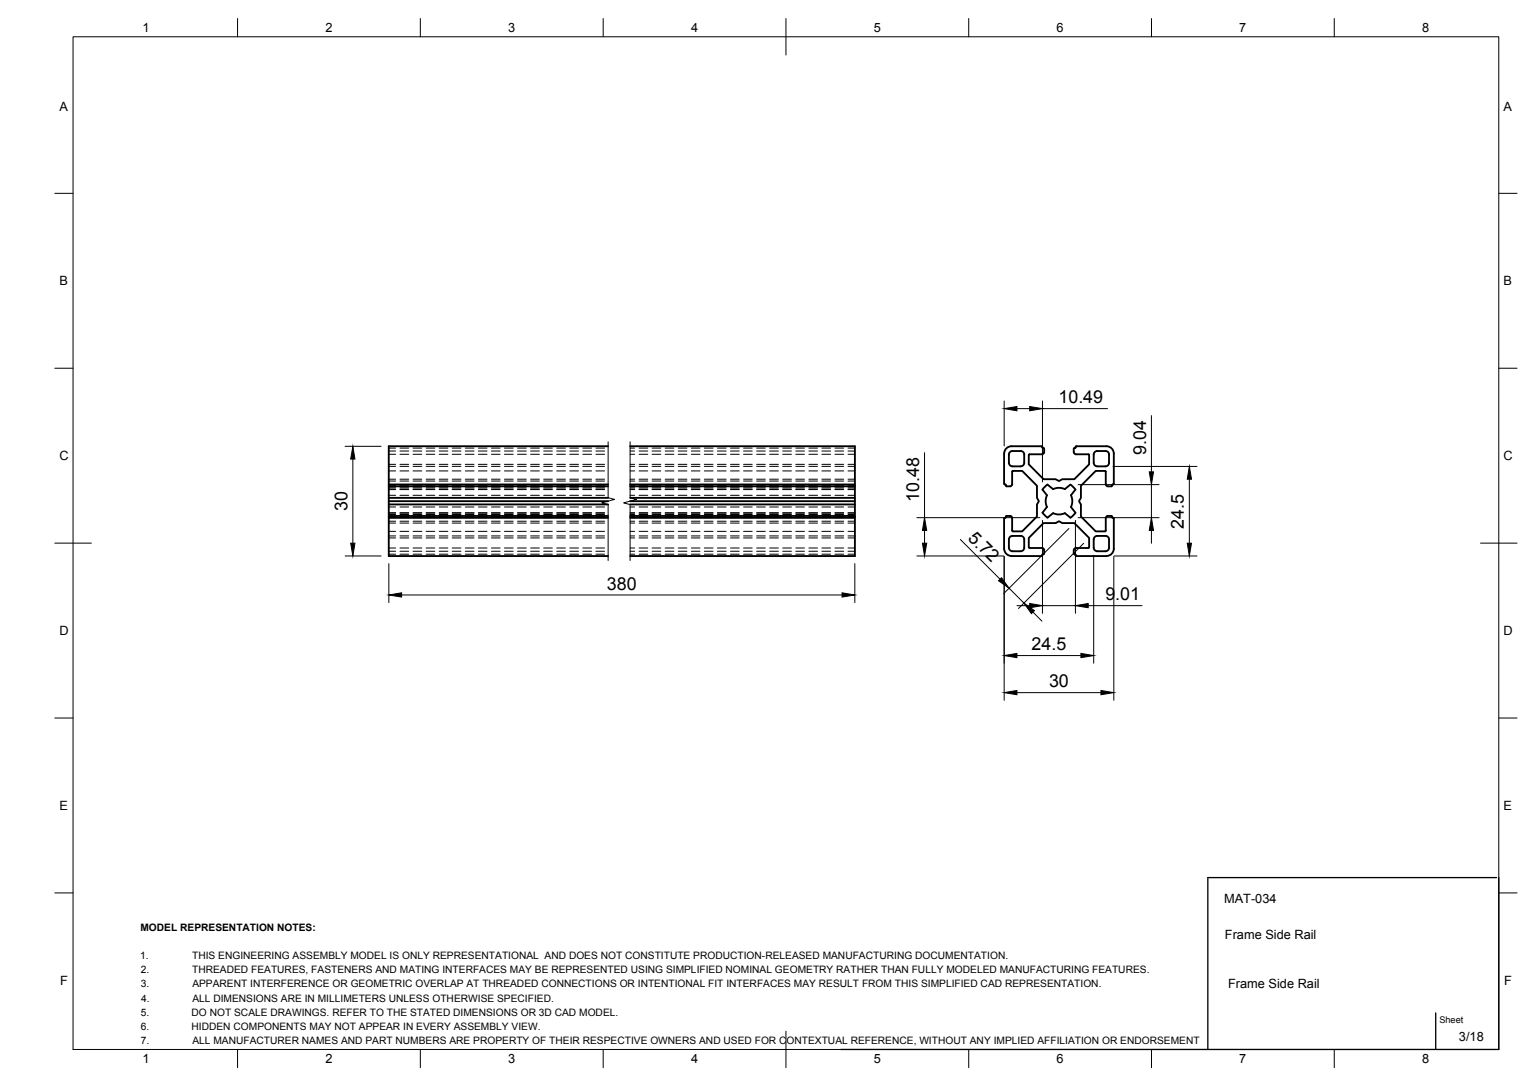
ISO-10303-21;
HEADER;
/* Generated by software containing ST-Developer
 * from STEP Tools, Inc. (www.steptools.com) 
 */

FILE_DESCRIPTION(
/* description */ ('STEP AP214'),
/* implementation_level */ '2;1');

FILE_NAME(
/* name */ 'Frame Side Rail.step',
/* time_stamp */ '2026-11-14T09:24:36-08:00',
/* author */ (''),
/* organization */ (''),
/* preprocessor_version */ 'ST-DEVELOPER v20.2',
/* originating_system */ 'Autodesk Translation Framework v15.17.0.0',
/* authorisation */ '');

FILE_SCHEMA (('AUTOMOTIVE_DESIGN { 1 0 10303 214 3 1 1 }'));
ENDSEC;

DATA;
#10=MECHANICAL_DESIGN_GEOMETRIC_PRESENTATION_REPRESENTATION('',(#213),#18867);
#181=SHAPE_REPRESENTATION_RELATIONSHIP('SRR','None',#18945,#197);
#197=ADVANCED_BREP_SHAPE_REPRESENTATION('',(#237),#18861);
#213=STYLED_ITEM('',(#19024),#237);
#237=MANIFOLD_SOLID_BREP('Body1',#10968);
#346=FACE_BOUND('',#1719,.T.);
#347=FACE_BOUND('',#1720,.T.);
#348=FACE_BOUND('',#1721,.T.);
#349=FACE_BOUND('',#1722,.T.);
#350=FACE_BOUND('',#1723,.T.);
#351=FACE_BOUND('',#1725,.T.);
#352=FACE_BOUND('',#1726,.T.);
#353=FACE_BOUND('',#1727,.T.);
#354=FACE_BOUND('',#1728,.T.);
#355=FACE_BOUND('',#1729,.T.);
#568=PLANE('',#11716);
#569=PLANE('',#11784);
#570=PLANE('',#11852);
#571=PLANE('',#11853);
#572=PLANE('',#11854);
#573=PLANE('',#11855);
#574=PLANE('',#11856);
#575=PLANE('',#11858);
#576=PLANE('',#11860);
#577=PLANE('',#11862);
#578=PLANE('',#11864);
#579=PLANE('',#11866);
#580=PLANE('',#11868);
#581=PLANE('',#11870);
#582=PLANE('',#11872);
#583=PLANE('',#11874);
#584=PLANE('',#11876);
#585=PLANE('',#11878);
#586=PLANE('',#11879);
#587=PLANE('',#11880);
#588=PLANE('',#11881);
#589=PLANE('',#11882);
#590=PLANE('',#11883);
#591=PLANE('',#11884);
#592=PLANE('',#11885);
#593=PLANE('',#11887);
#594=PLANE('',#11889);
#595=PLANE('',#11891);
#596=PLANE('',#11893);
#597=PLANE('',#11895);
#598=PLANE('',#11897);
#599=PLANE('',#11899);
#600=PLANE('',#11901);
#601=PLANE('',#11903);
#602=PLANE('',#11905);
#603=PLANE('',#11907);
#604=PLANE('',#11908);
#605=PLANE('',#11909);
#606=PLANE('',#11910);
#607=PLANE('',#11911);
#608=PLANE('',#11912);
#609=PLANE('',#11913);
#610=PLANE('',#11914);
#611=PLANE('',#11916);
#612=PLANE('',#11918);
#613=PLANE('',#11920);
#614=PLANE('',#11922);
#615=PLANE('',#11924);
#616=PLANE('',#11926);
#617=PLANE('',#11928);
#618=PLANE('',#11930);
#619=PLANE('',#11932);
#620=PLANE('',#11934);
#621=PLANE('',#11936);
#622=PLANE('',#11937);
#623=PLANE('',#11938);
#624=PLANE('',#11939);
#625=PLANE('',#11940);
#626=PLANE('',#11941);
#627=PLANE('',#11942);
#628=PLANE('',#11943);
#629=PLANE('',#11945);
#630=PLANE('',#11947);
#631=PLANE('',#11949);
#632=PLANE('',#11951);
#633=PLANE('',#11953);
#634=PLANE('',#11955);
#635=PLANE('',#11957);
#636=PLANE('',#11959);
#637=PLANE('',#11961);
#638=PLANE('',#11963);
#639=PLANE('',#11965);
#640=PLANE('',#11966);
#641=PLANE('',#11967);
#642=PLANE('',#11969);
#643=PLANE('',#11971);
#644=PLANE('',#11973);
#645=PLANE('',#11975);
#646=PLANE('',#11977);
#647=PLANE('',#11979);
#648=PLANE('',#11980);
#649=PLANE('',#11982);
#650=PLANE('',#11984);
#651=PLANE('',#11986);
#652=PLANE('',#11988);
#653=PLANE('',#11990);
#654=PLANE('',#11992);
#655=PLANE('',#11994);
#656=PLANE('',#11996);
#657=PLANE('',#11998);
#658=PLANE('',#12000);
#659=PLANE('',#12002);
#660=PLANE('',#12004);
#661=PLANE('',#12006);
#662=PLANE('',#12008);
#663=PLANE('',#12010);
#664=PLANE('',#12012);
#665=PLANE('',#12014);
#1026=FACE_OUTER_BOUND('',#1717,.T.);
#1027=FACE_OUTER_BOUND('',#1718,.T.);
#1028=FACE_OUTER_BOUND('',#1724,.T.);
#1029=FACE_OUTER_BOUND('',#1730,.T.);
#1030=FACE_OUTER_BOUND('',#1731,.T.);
#1031=FACE_OUTER_BOUND('',#1732,.T.);
#1032=FACE_OUTER_BOUND('',#1733,.T.);
#1033=FACE_OUTER_BOUND('',#1734,.T.);
#1034=FACE_OUTER_BOUND('',#1735,.T.);
#1035=FACE_OUTER_BOUND('',#1736,.T.);
#1036=FACE_OUTER_BOUND('',#1737,.T.);
#1037=FACE_OUTER_BOUND('',#1738,.T.);
#1038=FACE_OUTER_BOUND('',#1739,.T.);
#1039=FACE_OUTER_BOUND('',#1740,.T.);
#1040=FACE_OUTER_BOUND('',#1741,.T.);
#1041=FACE_OUTER_BOUND('',#1742,.T.);
#1042=FACE_OUTER_BOUND('',#1743,.T.);
#1043=FACE_OUTER_BOUND('',#1744,.T.);
#1044=FACE_OUTER_BOUND('',#1745,.T.);
#1045=FACE_OUTER_BOUND('',#1746,.T.);
#1046=FACE_OUTER_BOUND('',#1747,.T.);
#1047=FACE_OUTER_BOUND('',#1748,.T.);
#1048=FACE_OUTER_BOUND('',#1749,.T.);
#1049=FACE_OUTER_BOUND('',#1750,.T.);
#1050=FACE_OUTER_BOUND('',#1751,.T.);
#1051=FACE_OUTER_BOUND('',#1752,.T.);
#1052=FACE_OUTER_BOUND('',#1753,.T.);
#1053=FACE_OUTER_BOUND('',#1754,.T.);
#1054=FACE_OUTER_BOUND('',#1755,.T.);
#1055=FACE_OUTER_BOUND('',#1756,.T.);
#1056=FACE_OUTER_BOUND('',#1757,.T.);
#1057=FACE_OUTER_BOUND('',#1758,.T.);
#1058=FACE_OUTER_BOUND('',#1759,.T.);
#1059=FACE_OUTER_BOUND('',#1760,.T.);
#1060=FACE_OUTER_BOUND('',#1761,.T.);
#1061=FACE_OUTER_BOUND('',#1762,.T.);
#1062=FACE_OUTER_BOUND('',#1763,.T.);
#1063=FACE_OUTER_BOUND('',#1764,.T.);
#1064=FACE_OUTER_BOUND('',#1765,.T.);
#1065=FACE_OUTER_BOUND('',#1766,.T.);
#1066=FACE_OUTER_BOUND('',#1767,.T.);
#1067=FACE_OUTER_BOUND('',#1768,.T.);
#1068=FACE_OUTER_BOUND('',#1769,.T.);
#1069=FACE_OUTER_BOUND('',#1770,.T.);
#1070=FACE_OUTER_BOUND('',#1771,.T.);
#1071=FACE_OUTER_BOUND('',#1772,.T.);
#1072=FACE_OUTER_BOUND('',#1773,.T.);
#1073=FACE_OUTER_BOUND('',#1774,.T.);
#1074=FACE_OUTER_BOUND('',#1775,.T.);
#1075=FACE_OUTER_BOUND('',#1776,.T.);
#1076=FACE_OUTER_BOUND('',#1777,.T.);
#1077=FACE_OUTER_BOUND('',#1778,.T.);
#1078=FACE_OUTER_BOUND('',#1779,.T.);
#1079=FACE_OUTER_BOUND('',#1780,.T.);
#1080=FACE_OUTER_BOUND('',#1781,.T.);
#1081=FACE_OUTER_BOUND('',#1782,.T.);
#1082=FACE_OUTER_BOUND('',#1783,.T.);
#1083=FACE_OUTER_BOUND('',#1784,.T.);
#1084=FACE_OUTER_BOUND('',#1785,.T.);
#1085=FACE_OUTER_BOUND('',#1786,.T.);
#1086=FACE_OUTER_BOUND('',#1787,.T.);
#1087=FACE_OUTER_BOUND('',#1788,.T.);
#1088=FACE_OUTER_BOUND('',#1789,.T.);
#1089=FACE_OUTER_BOUND('',#1790,.T.);
#1090=FACE_OUTER_BOUND('',#1791,.T.);
#1091=FACE_OUTER_BOUND('',#1792,.T.);
#1092=FACE_OUTER_BOUND('',#1793,.T.);
#1093=FACE_OUTER_BOUND('',#1794,.T.);
#1094=FACE_OUTER_BOUND('',#1795,.T.);
#1095=FACE_OUTER_BOUND('',#1796,.T.);
#1096=FACE_OUTER_BOUND('',#1797,.T.);
#1097=FACE_OUTER_BOUND('',#1798,.T.);
#1098=FACE_OUTER_BOUND('',#1799,.T.);
#1099=FACE_OUTER_BOUND('',#1800,.T.);
#1100=FACE_OUTER_BOUND('',#1801,.T.);
#1101=FACE_OUTER_BOUND('',#1802,.T.);
#1102=FACE_OUTER_BOUND('',#1803,.T.);
#1103=FACE_OUTER_BOUND('',#1804,.T.);
#1104=FACE_OUTER_BOUND('',#1805,.T.);
#1105=FACE_OUTER_BOUND('',#1806,.T.);
#1106=FACE_OUTER_BOUND('',#1807,.T.);
#1107=FACE_OUTER_BOUND('',#1808,.T.);
#1108=FACE_OUTER_BOUND('',#1809,.T.);
#1109=FACE_OUTER_BOUND('',#1810,.T.);
#1110=FACE_OUTER_BOUND('',#1811,.T.);
#1111=FACE_OUTER_BOUND('',#1812,.T.);
#1112=FACE_OUTER_BOUND('',#1813,.T.);
#1113=FACE_OUTER_BOUND('',#1814,.T.);
#1114=FACE_OUTER_BOUND('',#1815,.T.);
#1115=FACE_OUTER_BOUND('',#1816,.T.);
#1116=FACE_OUTER_BOUND('',#1817,.T.);
#1117=FACE_OUTER_BOUND('',#1818,.T.);
#1118=FACE_OUTER_BOUND('',#1819,.T.);
#1119=FACE_OUTER_BOUND('',#1820,.T.);
#1120=FACE_OUTER_BOUND('',#1821,.T.);
#1121=FACE_OUTER_BOUND('',#1822,.T.);
#1122=FACE_OUTER_BOUND('',#1823,.T.);
#1123=FACE_OUTER_BOUND('',#1824,.T.);
#1124=FACE_OUTER_BOUND('',#1825,.T.);
#1125=FACE_OUTER_BOUND('',#1826,.T.);
#1126=FACE_OUTER_BOUND('',#1827,.T.);
#1127=FACE_OUTER_BOUND('',#1828,.T.);
#1128=FACE_OUTER_BOUND('',#1829,.T.);
#1129=FACE_OUTER_BOUND('',#1830,.T.);
#1130=FACE_OUTER_BOUND('',#1831,.T.);
#1131=FACE_OUTER_BOUND('',#1832,.T.);
#1132=FACE_OUTER_BOUND('',#1833,.T.);
#1133=FACE_OUTER_BOUND('',#1834,.T.);
#1134=FACE_OUTER_BOUND('',#1835,.T.);
#1135=FACE_OUTER_BOUND('',#1836,.T.);
#1136=FACE_OUTER_BOUND('',#1837,.T.);
#1137=FACE_OUTER_BOUND('',#1838,.T.);
#1138=FACE_OUTER_BOUND('',#1839,.T.);
#1139=FACE_OUTER_BOUND('',#1840,.T.);
#1140=FACE_OUTER_BOUND('',#1841,.T.);
#1141=FACE_OUTER_BOUND('',#1842,.T.);
#1142=FACE_OUTER_BOUND('',#1843,.T.);
#1143=FACE_OUTER_BOUND('',#1844,.T.);
#1144=FACE_OUTER_BOUND('',#1845,.T.);
#1145=FACE_OUTER_BOUND('',#1846,.T.);
#1146=FACE_OUTER_BOUND('',#1847,.T.);
#1147=FACE_OUTER_BOUND('',#1848,.T.);
#1148=FACE_OUTER_BOUND('',#1849,.T.);
#1149=FACE_OUTER_BOUND('',#1850,.T.);
#1150=FACE_OUTER_BOUND('',#1851,.T.);
#1151=FACE_OUTER_BOUND('',#1852,.T.);
#1152=FACE_OUTER_BOUND('',#1853,.T.);
#1153=FACE_OUTER_BOUND('',#1854,.T.);
#1154=FACE_OUTER_BOUND('',#1855,.T.);
#1155=FACE_OUTER_BOUND('',#1856,.T.);
#1156=FACE_OUTER_BOUND('',#1857,.T.);
#1157=FACE_OUTER_BOUND('',#1858,.T.);
#1158=FACE_OUTER_BOUND('',#1859,.T.);
#1159=FACE_OUTER_BOUND('',#1860,.T.);
#1160=FACE_OUTER_BOUND('',#1861,.T.);
#1161=FACE_OUTER_BOUND('',#1862,.T.);
#1162=FACE_OUTER_BOUND('',#1863,.T.);
#1163=FACE_OUTER_BOUND('',#1864,.T.);
#1164=FACE_OUTER_BOUND('',#1865,.T.);
#1165=FACE_OUTER_BOUND('',#1866,.T.);
#1166=FACE_OUTER_BOUND('',#1867,.T.);
#1167=FACE_OUTER_BOUND('',#1868,.T.);
#1168=FACE_OUTER_BOUND('',#1869,.T.);
#1169=FACE_OUTER_BOUND('',#1870,.T.);
#1170=FACE_OUTER_BOUND('',#1871,.T.);
#1171=FACE_OUTER_BOUND('',#1872,.T.);
#1172=FACE_OUTER_BOUND('',#1873,.T.);
#1173=FACE_OUTER_BOUND('',#1874,.T.);
#1174=FACE_OUTER_BOUND('',#1875,.T.);
#1175=FACE_OUTER_BOUND('',#1876,.T.);
#1176=FACE_OUTER_BOUND('',#1877,.T.);
#1177=FACE_OUTER_BOUND('',#1878,.T.);
#1178=FACE_OUTER_BOUND('',#1879,.T.);
#1179=FACE_OUTER_BOUND('',#1880,.T.);
#1180=FACE_OUTER_BOUND('',#1881,.T.);
#1181=FACE_OUTER_BOUND('',#1882,.T.);
#1182=FACE_OUTER_BOUND('',#1883,.T.);
#1183=FACE_OUTER_BOUND('',#1884,.T.);
#1184=FACE_OUTER_BOUND('',#1885,.T.);
#1185=FACE_OUTER_BOUND('',#1886,.T.);
#1186=FACE_OUTER_BOUND('',#1887,.T.);
#1187=FACE_OUTER_BOUND('',#1888,.T.);
#1188=FACE_OUTER_BOUND('',#1889,.T.);
#1189=FACE_OUTER_BOUND('',#1890,.T.);
#1190=FACE_OUTER_BOUND('',#1891,.T.);
#1191=FACE_OUTER_BOUND('',#1892,.T.);
#1717=EDGE_LOOP('',(#8580,#8581,#8582,#8583));
#1718=EDGE_LOOP('',(#8584,#8585,#8586,#8587,#8588,#8589,#8590,#8591,#8592,
#8593,#8594,#8595,#8596,#8597,#8598,#8599,#8600,#8601,#8602,#8603,#8604,
#8605,#8606,#8607,#8608,#8609,#8610,#8611,#8612,#8613,#8614,#8615,#8616,
#8617,#8618,#8619,#8620,#8621,#8622,#8623,#8624,#8625,#8626,#8627,#8628,
#8629,#8630,#8631,#8632,#8633,#8634,#8635,#8636,#8637,#8638,#8639,#8640,
#8641,#8642,#8643,#8644,#8645,#8646,#8647,#8648,#8649,#8650,#8651,#8652,
#8653,#8654,#8655,#8656,#8657,#8658,#8659,#8660,#8661,#8662,#8663,#8664,
#8665,#8666,#8667,#8668,#8669,#8670,#8671,#8672,#8673,#8674,#8675,#8676,
#8677,#8678,#8679,#8680,#8681,#8682,#8683,#8684,#8685,#8686,#8687,#8688,
#8689,#8690,#8691,#8692,#8693,#8694,#8695,#8696,#8697,#8698,#8699));
#1719=EDGE_LOOP('',(#8700,#8701,#8702,#8703,#8704,#8705,#8706,#8707));
#1720=EDGE_LOOP('',(#8708,#8709,#8710,#8711,#8712,#8713,#8714,#8715,#8716,
#8717,#8718,#8719,#8720,#8721,#8722,#8723));
#1721=EDGE_LOOP('',(#8724,#8725,#8726,#8727,#8728,#8729,#8730,#8731));
#1722=EDGE_LOOP('',(#8732,#8733,#8734,#8735,#8736,#8737,#8738,#8739));
#1723=EDGE_LOOP('',(#8740,#8741,#8742,#8743,#8744,#8745,#8746,#8747));
#1724=EDGE_LOOP('',(#8748,#8749,#8750,#8751,#8752,#8753,#8754,#8755,#8756,
#8757,#8758,#8759,#8760,#8761,#8762,#8763,#8764,#8765,#8766,#8767,#8768,
#8769,#8770,#8771,#8772,#8773,#8774,#8775,#8776,#8777,#8778,#8779,#8780,
#8781,#8782,#8783,#8784,#8785,#8786,#8787,#8788,#8789,#8790,#8791,#8792,
#8793,#8794,#8795,#8796,#8797,#8798,#8799,#8800,#8801,#8802,#8803,#8804,
#8805,#8806,#8807,#8808,#8809,#8810,#8811,#8812,#8813,#8814,#8815,#8816,
#8817,#8818,#8819,#8820,#8821,#8822,#8823,#8824,#8825,#8826,#8827,#8828,
#8829,#8830,#8831,#8832,#8833,#8834,#8835,#8836,#8837,#8838,#8839,#8840,
#8841,#8842,#8843,#8844,#8845,#8846,#8847,#8848,#8849,#8850,#8851,#8852,
#8853,#8854,#8855,#8856,#8857,#8858,#8859,#8860,#8861,#8862,#8863));
#1725=EDGE_LOOP('',(#8864,#8865,#8866,#8867,#8868,#8869,#8870,#8871));
#1726=EDGE_LOOP('',(#8872,#8873,#8874,#8875,#8876,#8877,#8878,#8879));
#1727=EDGE_LOOP('',(#8880,#8881,#8882,#8883,#8884,#8885,#8886,#8887));
#1728=EDGE_LOOP('',(#8888,#8889,#8890,#8891,#8892,#8893,#8894,#8895));
#1729=EDGE_LOOP('',(#8896,#8897,#8898,#8899,#8900,#8901,#8902,#8903,#8904,
#8905,#8906,#8907,#8908,#8909,#8910,#8911));
#1730=EDGE_LOOP('',(#8912,#8913,#8914,#8915));
#1731=EDGE_LOOP('',(#8916,#8917,#8918,#8919));
#1732=EDGE_LOOP('',(#8920,#8921,#8922,#8923));
#1733=EDGE_LOOP('',(#8924,#8925,#8926,#8927));
#1734=EDGE_LOOP('',(#8928,#8929,#8930,#8931));
#1735=EDGE_LOOP('',(#8932,#8933,#8934,#8935));
#1736=EDGE_LOOP('',(#8936,#8937,#8938,#8939));
#1737=EDGE_LOOP('',(#8940,#8941,#8942,#8943));
#1738=EDGE_LOOP('',(#8944,#8945,#8946,#8947));
#1739=EDGE_LOOP('',(#8948,#8949,#8950,#8951));
#1740=EDGE_LOOP('',(#8952,#8953,#8954,#8955));
#1741=EDGE_LOOP('',(#8956,#8957,#8958,#8959));
#1742=EDGE_LOOP('',(#8960,#8961,#8962,#8963));
#1743=EDGE_LOOP('',(#8964,#8965,#8966,#8967));
#1744=EDGE_LOOP('',(#8968,#8969,#8970,#8971));
#1745=EDGE_LOOP('',(#8972,#8973,#8974,#8975));
#1746=EDGE_LOOP('',(#8976,#8977,#8978,#8979));
#1747=EDGE_LOOP('',(#8980,#8981,#8982,#8983));
#1748=EDGE_LOOP('',(#8984,#8985,#8986,#8987));
#1749=EDGE_LOOP('',(#8988,#8989,#8990,#8991));
#1750=EDGE_LOOP('',(#8992,#8993,#8994,#8995));
#1751=EDGE_LOOP('',(#8996,#8997,#8998,#8999));
#1752=EDGE_LOOP('',(#9000,#9001,#9002,#9003));
#1753=EDGE_LOOP('',(#9004,#9005,#9006,#9007));
#1754=EDGE_LOOP('',(#9008,#9009,#9010,#9011));
#1755=EDGE_LOOP('',(#9012,#9013,#9014,#9015));
#1756=EDGE_LOOP('',(#9016,#9017,#9018,#9019));
#1757=EDGE_LOOP('',(#9020,#9021,#9022,#9023));
#1758=EDGE_LOOP('',(#9024,#9025,#9026,#9027));
#1759=EDGE_LOOP('',(#9028,#9029,#9030,#9031));
#1760=EDGE_LOOP('',(#9032,#9033,#9034,#9035));
#1761=EDGE_LOOP('',(#9036,#9037,#9038,#9039));
#1762=EDGE_LOOP('',(#9040,#9041,#9042,#9043));
#1763=EDGE_LOOP('',(#9044,#9045,#9046,#9047));
#1764=EDGE_LOOP('',(#9048,#9049,#9050,#9051));
#1765=EDGE_LOOP('',(#9052,#9053,#9054,#9055));
#1766=EDGE_LOOP('',(#9056,#9057,#9058,#9059));
#1767=EDGE_LOOP('',(#9060,#9061,#9062,#9063));
#1768=EDGE_LOOP('',(#9064,#9065,#9066,#9067));
#1769=EDGE_LOOP('',(#9068,#9069,#9070,#9071));
#1770=EDGE_LOOP('',(#9072,#9073,#9074,#9075));
#1771=EDGE_LOOP('',(#9076,#9077,#9078,#9079));
#1772=EDGE_LOOP('',(#9080,#9081,#9082,#9083));
#1773=EDGE_LOOP('',(#9084,#9085,#9086,#9087));
#1774=EDGE_LOOP('',(#9088,#9089,#9090,#9091));
#1775=EDGE_LOOP('',(#9092,#9093,#9094,#9095));
#1776=EDGE_LOOP('',(#9096,#9097,#9098,#9099));
#1777=EDGE_LOOP('',(#9100,#9101,#9102,#9103));
#1778=EDGE_LOOP('',(#9104,#9105,#9106,#9107));
#1779=EDGE_LOOP('',(#9108,#9109,#9110,#9111));
#1780=EDGE_LOOP('',(#9112,#9113,#9114,#9115));
#1781=EDGE_LOOP('',(#9116,#9117,#9118,#9119));
#1782=EDGE_LOOP('',(#9120,#9121,#9122,#9123));
#1783=EDGE_LOOP('',(#9124,#9125,#9126,#9127));
#1784=EDGE_LOOP('',(#9128,#9129,#9130,#9131));
#1785=EDGE_LOOP('',(#9132,#9133,#9134,#9135));
#1786=EDGE_LOOP('',(#9136,#9137,#9138,#9139));
#1787=EDGE_LOOP('',(#9140,#9141,#9142,#9143));
#1788=EDGE_LOOP('',(#9144,#9145,#9146,#9147));
#1789=EDGE_LOOP('',(#9148,#9149,#9150,#9151));
#1790=EDGE_LOOP('',(#9152,#9153,#9154,#9155));
#1791=EDGE_LOOP('',(#9156,#9157,#9158,#9159));
#1792=EDGE_LOOP('',(#9160,#9161,#9162,#9163));
#1793=EDGE_LOOP('',(#9164,#9165,#9166,#9167));
#1794=EDGE_LOOP('',(#9168,#9169,#9170,#9171));
#1795=EDGE_LOOP('',(#9172,#9173,#9174,#9175));
#1796=EDGE_LOOP('',(#9176,#9177,#9178,#9179));
#1797=EDGE_LOOP('',(#9180,#9181,#9182,#9183));
#1798=EDGE_LOOP('',(#9184,#9185,#9186,#9187));
#1799=EDGE_LOOP('',(#9188,#9189,#9190,#9191));
#1800=EDGE_LOOP('',(#9192,#9193,#9194,#9195));
#1801=EDGE_LOOP('',(#9196,#9197,#9198,#9199));
#1802=EDGE_LOOP('',(#9200,#9201,#9202,#9203));
#1803=EDGE_LOOP('',(#9204,#9205,#9206,#9207));
#1804=EDGE_LOOP('',(#9208,#9209,#9210,#9211));
#1805=EDGE_LOOP('',(#9212,#9213,#9214,#9215));
#1806=EDGE_LOOP('',(#9216,#9217,#9218,#9219));
#1807=EDGE_LOOP('',(#9220,#9221,#9222,#9223));
#1808=EDGE_LOOP('',(#9224,#9225,#9226,#9227));
#1809=EDGE_LOOP('',(#9228,#9229,#9230,#9231));
#1810=EDGE_LOOP('',(#9232,#9233,#9234,#9235));
#1811=EDGE_LOOP('',(#9236,#9237,#9238,#9239));
#1812=EDGE_LOOP('',(#9240,#9241,#9242,#9243));
#1813=EDGE_LOOP('',(#9244,#9245,#9246,#9247));
#1814=EDGE_LOOP('',(#9248,#9249,#9250,#9251));
#1815=EDGE_LOOP('',(#9252,#9253,#9254,#9255));
#1816=EDGE_LOOP('',(#9256,#9257,#9258,#9259));
#1817=EDGE_LOOP('',(#9260,#9261,#9262,#9263));
#1818=EDGE_LOOP('',(#9264,#9265,#9266,#9267));
#1819=EDGE_LOOP('',(#9268,#9269,#9270,#9271));
#1820=EDGE_LOOP('',(#9272,#9273,#9274,#9275));
#1821=EDGE_LOOP('',(#9276,#9277,#9278,#9279));
#1822=EDGE_LOOP('',(#9280,#9281,#9282,#9283));
#1823=EDGE_LOOP('',(#9284,#9285,#9286,#9287));
#1824=EDGE_LOOP('',(#9288,#9289,#9290,#9291));
#1825=EDGE_LOOP('',(#9292,#9293,#9294,#9295));
#1826=EDGE_LOOP('',(#9296,#9297,#9298,#9299));
#1827=EDGE_LOOP('',(#9300,#9301,#9302,#9303));
#1828=EDGE_LOOP('',(#9304,#9305,#9306,#9307));
#1829=EDGE_LOOP('',(#9308,#9309,#9310,#9311));
#1830=EDGE_LOOP('',(#9312,#9313,#9314,#9315));
#1831=EDGE_LOOP('',(#9316,#9317,#9318,#9319));
#1832=EDGE_LOOP('',(#9320,#9321,#9322,#9323));
#1833=EDGE_LOOP('',(#9324,#9325,#9326,#9327));
#1834=EDGE_LOOP('',(#9328,#9329,#9330,#9331));
#1835=EDGE_LOOP('',(#9332,#9333,#9334,#9335));
#1836=EDGE_LOOP('',(#9336,#9337,#9338,#9339));
#1837=EDGE_LOOP('',(#9340,#9341,#9342,#9343));
#1838=EDGE_LOOP('',(#9344,#9345,#9346,#9347));
#1839=EDGE_LOOP('',(#9348,#9349,#9350,#9351));
#1840=EDGE_LOOP('',(#9352,#9353,#9354,#9355));
#1841=EDGE_LOOP('',(#9356,#9357,#9358,#9359));
#1842=EDGE_LOOP('',(#9360,#9361,#9362,#9363));
#1843=EDGE_LOOP('',(#9364,#9365,#9366,#9367));
#1844=EDGE_LOOP('',(#9368,#9369,#9370,#9371));
#1845=EDGE_LOOP('',(#9372,#9373,#9374,#9375));
#1846=EDGE_LOOP('',(#9376,#9377,#9378,#9379));
#1847=EDGE_LOOP('',(#9380,#9381,#9382,#9383));
#1848=EDGE_LOOP('',(#9384,#9385,#9386,#9387));
#1849=EDGE_LOOP('',(#9388,#9389,#9390,#9391));
#1850=EDGE_LOOP('',(#9392,#9393,#9394,#9395));
#1851=EDGE_LOOP('',(#9396,#9397,#9398,#9399));
#1852=EDGE_LOOP('',(#9400,#9401,#9402,#9403));
#1853=EDGE_LOOP('',(#9404,#9405,#9406,#9407));
#1854=EDGE_LOOP('',(#9408,#9409,#9410,#9411));
#1855=EDGE_LOOP('',(#9412,#9413,#9414,#9415));
#1856=EDGE_LOOP('',(#9416,#9417,#9418,#9419));
#1857=EDGE_LOOP('',(#9420,#9421,#9422,#9423));
#1858=EDGE_LOOP('',(#9424,#9425,#9426,#9427));
#1859=EDGE_LOOP('',(#9428,#9429,#9430,#9431));
#1860=EDGE_LOOP('',(#9432,#9433,#9434,#9435));
#1861=EDGE_LOOP('',(#9436,#9437,#9438,#9439));
#1862=EDGE_LOOP('',(#9440,#9441,#9442,#9443));
#1863=EDGE_LOOP('',(#9444,#9445,#9446,#9447));
#1864=EDGE_LOOP('',(#9448,#9449,#9450,#9451));
#1865=EDGE_LOOP('',(#9452,#9453,#9454,#9455));
#1866=EDGE_LOOP('',(#9456,#9457,#9458,#9459));
#1867=EDGE_LOOP('',(#9460,#9461,#9462,#9463));
#1868=EDGE_LOOP('',(#9464,#9465,#9466,#9467));
#1869=EDGE_LOOP('',(#9468,#9469,#9470,#9471));
#1870=EDGE_LOOP('',(#9472,#9473,#9474,#9475));
#1871=EDGE_LOOP('',(#9476,#9477,#9478,#9479));
#1872=EDGE_LOOP('',(#9480,#9481,#9482,#9483));
#1873=EDGE_LOOP('',(#9484,#9485,#9486,#9487));
#1874=EDGE_LOOP('',(#9488,#9489,#9490,#9491));
#1875=EDGE_LOOP('',(#9492,#9493,#9494,#9495));
#1876=EDGE_LOOP('',(#9496,#9497,#9498,#9499));
#1877=EDGE_LOOP('',(#9500,#9501,#9502,#9503));
#1878=EDGE_LOOP('',(#9504,#9505,#9506,#9507));
#1879=EDGE_LOOP('',(#9508,#9509,#9510,#9511));
#1880=EDGE_LOOP('',(#9512,#9513,#9514,#9515));
#1881=EDGE_LOOP('',(#9516,#9517,#9518,#9519));
#1882=EDGE_LOOP('',(#9520,#9521,#9522,#9523));
#1883=EDGE_LOOP('',(#9524,#9525,#9526,#9527));
#1884=EDGE_LOOP('',(#9528,#9529,#9530,#9531));
#1885=EDGE_LOOP('',(#9532,#9533,#9534,#9535));
#1886=EDGE_LOOP('',(#9536,#9537,#9538,#9539));
#1887=EDGE_LOOP('',(#9540,#9541,#9542,#9543));
#1888=EDGE_LOOP('',(#9544,#9545,#9546,#9547));
#1889=EDGE_LOOP('',(#9548,#9549,#9550,#9551));
#1890=EDGE_LOOP('',(#9552,#9553,#9554,#9555));
#1891=EDGE_LOOP('',(#9556,#9557,#9558,#9559));
#1892=EDGE_LOOP('',(#9560,#9561,#9562,#9563));
#2538=LINE('',#17197,#3552);
#2539=LINE('',#17200,#3553);
#2540=LINE('',#17204,#3554);
#2541=LINE('',#17206,#3555);
#2542=LINE('',#17208,#3556);
#2543=LINE('',#17210,#3557);
#2544=LINE('',#17212,#3558);
#2545=LINE('',#17216,#3559);
#2546=LINE('',#17220,#3560);
#2547=LINE('',#17224,#3561);
#2548=LINE('',#17228,#3562);
#2549=LINE('',#17232,#3563);
#2550=LINE('',#17236,#3564);
#2551=LINE('',#17240,#3565);
#2552=LINE('',#17244,#3566);
#2553=LINE('',#17248,#3567);
#2554=LINE('',#17252,#3568);
#2555=LINE('',#17256,#3569);
#2556=LINE('',#17258,#3570);
#2557=LINE('',#17260,#3571);
#2558=LINE('',#17262,#3572);
#2559=LINE('',#17264,#3573);
#2560=LINE('',#17266,#3574);
#2561=LINE('',#17268,#3575);
#2562=LINE('',#17270,#3576);
#2563=LINE('',#17274,#3577);
#2564=LINE('',#17278,#3578);
#2565=LINE('',#17282,#3579);
#2566=LINE('',#17286,#3580);
#2567=LINE('',#17290,#3581);
#2568=LINE('',#17294,#3582);
#2569=LINE('',#17298,#3583);
#2570=LINE('',#17302,#3584);
#2571=LINE('',#17306,#3585);
#2572=LINE('',#17310,#3586);
#2573=LINE('',#17314,#3587);
#2574=LINE('',#17316,#3588);
#2575=LINE('',#17318,#3589);
#2576=LINE('',#17320,#3590);
#2577=LINE('',#17322,#3591);
#2578=LINE('',#17324,#3592);
#2579=LINE('',#17326,#3593);
#2580=LINE('',#17328,#3594);
#2581=LINE('',#17332,#3595);
#2582=LINE('',#17336,#3596);
#2583=LINE('',#17340,#3597);
#2584=LINE('',#17344,#3598);
#2585=LINE('',#17348,#3599);
#2586=LINE('',#17352,#3600);
#2587=LINE('',#17356,#3601);
#2588=LINE('',#17360,#3602);
#2589=LINE('',#17364,#3603);
#2590=LINE('',#17368,#3604);
#2591=LINE('',#17372,#3605);
#2592=LINE('',#17374,#3606);
#2593=LINE('',#17376,#3607);
#2594=LINE('',#17378,#3608);
#2595=LINE('',#17380,#3609);
#2596=LINE('',#17382,#3610);
#2597=LINE('',#17384,#3611);
#2598=LINE('',#17386,#3612);
#2599=LINE('',#17390,#3613);
#2600=LINE('',#17394,#3614);
#2601=LINE('',#17398,#3615);
#2602=LINE('',#17402,#3616);
#2603=LINE('',#17406,#3617);
#2604=LINE('',#17410,#3618);
#2605=LINE('',#17414,#3619);
#2606=LINE('',#17418,#3620);
#2607=LINE('',#17422,#3621);
#2608=LINE('',#17426,#3622);
#2609=LINE('',#17430,#3623);
#2610=LINE('',#17432,#3624);
#2611=LINE('',#17433,#3625);
#2612=LINE('',#17436,#3626);
#2613=LINE('',#17440,#3627);
#2614=LINE('',#17444,#3628);
#2615=LINE('',#17448,#3629);
#2616=LINE('',#17452,#3630);
#2617=LINE('',#17456,#3631);
#2618=LINE('',#17460,#3632);
#2619=LINE('',#17464,#3633);
#2620=LINE('',#17468,#3634);
#2621=LINE('',#17472,#3635);
#2622=LINE('',#17475,#3636);
#2623=LINE('',#17477,#3637);
#2624=LINE('',#17481,#3638);
#2625=LINE('',#17485,#3639);
#2626=LINE('',#17489,#3640);
#2627=LINE('',#17493,#3641);
#2628=LINE('',#17497,#3642);
#2629=LINE('',#17501,#3643);
#2630=LINE('',#17505,#3644);
#2631=LINE('',#17509,#3645);
#2632=LINE('',#17513,#3646);
#2633=LINE('',#17517,#3647);
#2634=LINE('',#17521,#3648);
#2635=LINE('',#17525,#3649);
#2636=LINE('',#17530,#3650);
#2637=LINE('',#17532,#3651);
#2638=LINE('',#17534,#3652);
#2639=LINE('',#17536,#3653);
#2640=LINE('',#17540,#3654);
#2641=LINE('',#17544,#3655);
#2642=LINE('',#17548,#3656);
#2643=LINE('',#17552,#3657);
#2644=LINE('',#17556,#3658);
#2645=LINE('',#17560,#3659);
#2646=LINE('',#17564,#3660);
#2647=LINE('',#17568,#3661);
#2648=LINE('',#17572,#3662);
#2649=LINE('',#17576,#3663);
#2650=LINE('',#17580,#3664);
#2651=LINE('',#17582,#3665);
#2652=LINE('',#17584,#3666);
#2653=LINE('',#17586,#3667);
#2654=LINE('',#17588,#3668);
#2655=LINE('',#17590,#3669);
#2656=LINE('',#17592,#3670);
#2657=LINE('',#17594,#3671);
#2658=LINE('',#17598,#3672);
#2659=LINE('',#17602,#3673);
#2660=LINE('',#17606,#3674);
#2661=LINE('',#17610,#3675);
#2662=LINE('',#17614,#3676);
#2663=LINE('',#17618,#3677);
#2664=LINE('',#17622,#3678);
#2665=LINE('',#17626,#3679);
#2666=LINE('',#17630,#3680);
#2667=LINE('',#17634,#3681);
#2668=LINE('',#17638,#3682);
#2669=LINE('',#17640,#3683);
#2670=LINE('',#17642,#3684);
#2671=LINE('',#17644,#3685);
#2672=LINE('',#17646,#3686);
#2673=LINE('',#17648,#3687);
#2674=LINE('',#17650,#3688);
#2675=LINE('',#17652,#3689);
#2676=LINE('',#17656,#3690);
#2677=LINE('',#17660,#3691);
#2678=LINE('',#17664,#3692);
#2679=LINE('',#17668,#3693);
#2680=LINE('',#17672,#3694);
#2681=LINE('',#17676,#3695);
#2682=LINE('',#17680,#3696);
#2683=LINE('',#17684,#3697);
#2684=LINE('',#17688,#3698);
#2685=LINE('',#17692,#3699);
#2686=LINE('',#17696,#3700);
#2687=LINE('',#17698,#3701);
#2688=LINE('',#17700,#3702);
#2689=LINE('',#17702,#3703);
#2690=LINE('',#17704,#3704);
#2691=LINE('',#17706,#3705);
#2692=LINE('',#17708,#3706);
#2693=LINE('',#17710,#3707);
#2694=LINE('',#17714,#3708);
#2695=LINE('',#17718,#3709);
#2696=LINE('',#17722,#3710);
#2697=LINE('',#17726,#3711);
#2698=LINE('',#17730,#3712);
#2699=LINE('',#17734,#3713);
#2700=LINE('',#17738,#3714);
#2701=LINE('',#17742,#3715);
#2702=LINE('',#17746,#3716);
#2703=LINE('',#17750,#3717);
#2704=LINE('',#17754,#3718);
#2705=LINE('',#17756,#3719);
#2706=LINE('',#17758,#3720);
#2707=LINE('',#17759,#3721);
#2708=LINE('',#17764,#3722);
#2709=LINE('',#17768,#3723);
#2710=LINE('',#17772,#3724);
#2711=LINE('',#17775,#3725);
#2712=LINE('',#17780,#3726);
#2713=LINE('',#17784,#3727);
#2714=LINE('',#17788,#3728);
#2715=LINE('',#17791,#3729);
#2716=LINE('',#17796,#3730);
#2717=LINE('',#17800,#3731);
#2718=LINE('',#17804,#3732);
#2719=LINE('',#17807,#3733);
#2720=LINE('',#17812,#3734);
#2721=LINE('',#17816,#3735);
#2722=LINE('',#17820,#3736);
#2723=LINE('',#17823,#3737);
#2724=LINE('',#17828,#3738);
#2725=LINE('',#17831,#3739);
#2726=LINE('',#17833,#3740);
#2727=LINE('',#17837,#3741);
#2728=LINE('',#17841,#3742);
#2729=LINE('',#17845,#3743);
#2730=LINE('',#17849,#3744);
#2731=LINE('',#17852,#3745);
#2732=LINE('',#17854,#3746);
#2733=LINE('',#17855,#3747);
#2734=LINE('',#17857,#3748);
#2735=LINE('',#17859,#3749);
#2736=LINE('',#17861,#3750);
#2737=LINE('',#17863,#3751);
#2738=LINE('',#17865,#3752);
#2739=LINE('',#17867,#3753);
#2740=LINE('',#17869,#3754);
#2741=LINE('',#17871,#3755);
#2742=LINE('',#17873,#3756);
#2743=LINE('',#17875,#3757);
#2744=LINE('',#17877,#3758);
#2745=LINE('',#17879,#3759);
#2746=LINE('',#17881,#3760);
#2747=LINE('',#17883,#3761);
#2748=LINE('',#17885,#3762);
#2749=LINE('',#17887,#3763);
#2750=LINE('',#17889,#3764);
#2751=LINE('',#17891,#3765);
#2752=LINE('',#17893,#3766);
#2753=LINE('',#17895,#3767);
#2754=LINE('',#17897,#3768);
#2755=LINE('',#17899,#3769);
#2756=LINE('',#17901,#3770);
#2757=LINE('',#17903,#3771);
#2758=LINE('',#17905,#3772);
#2759=LINE('',#17907,#3773);
#2760=LINE('',#17909,#3774);
#2761=LINE('',#17911,#3775);
#2762=LINE('',#17913,#3776);
#2763=LINE('',#17915,#3777);
#2764=LINE('',#17917,#3778);
#2765=LINE('',#17919,#3779);
#2766=LINE('',#17921,#3780);
#2767=LINE('',#17923,#3781);
#2768=LINE('',#17925,#3782);
#2769=LINE('',#17927,#3783);
#2770=LINE('',#17929,#3784);
#2771=LINE('',#17931,#3785);
#2772=LINE('',#17933,#3786);
#2773=LINE('',#17935,#3787);
#2774=LINE('',#17937,#3788);
#2775=LINE('',#17939,#3789);
#2776=LINE('',#17941,#3790);
#2777=LINE('',#17943,#3791);
#2778=LINE('',#17945,#3792);
#2779=LINE('',#17947,#3793);
#2780=LINE('',#17949,#3794);
#2781=LINE('',#17951,#3795);
#2782=LINE('',#17953,#3796);
#2783=LINE('',#17955,#3797);
#2784=LINE('',#17957,#3798);
#2785=LINE('',#17959,#3799);
#2786=LINE('',#17961,#3800);
#2787=LINE('',#17963,#3801);
#2788=LINE('',#17965,#3802);
#2789=LINE('',#17967,#3803);
#2790=LINE('',#17969,#3804);
#2791=LINE('',#17971,#3805);
#2792=LINE('',#17973,#3806);
#2793=LINE('',#17975,#3807);
#2794=LINE('',#17977,#3808);
#2795=LINE('',#17979,#3809);
#2796=LINE('',#17981,#3810);
#2797=LINE('',#17983,#3811);
#2798=LINE('',#17985,#3812);
#2799=LINE('',#17987,#3813);
#2800=LINE('',#17989,#3814);
#2801=LINE('',#17991,#3815);
#2802=LINE('',#17993,#3816);
#2803=LINE('',#17995,#3817);
#2804=LINE('',#17997,#3818);
#2805=LINE('',#17999,#3819);
#2806=LINE('',#18001,#3820);
#2807=LINE('',#18003,#3821);
#2808=LINE('',#18005,#3822);
#2809=LINE('',#18007,#3823);
#2810=LINE('',#18009,#3824);
#2811=LINE('',#18011,#3825);
#2812=LINE('',#18013,#3826);
#2813=LINE('',#18015,#3827);
#2814=LINE('',#18017,#3828);
#2815=LINE('',#18019,#3829);
#2816=LINE('',#18021,#3830);
#2817=LINE('',#18023,#3831);
#2818=LINE('',#18025,#3832);
#2819=LINE('',#18027,#3833);
#2820=LINE('',#18029,#3834);
#2821=LINE('',#18031,#3835);
#2822=LINE('',#18033,#3836);
#2823=LINE('',#18035,#3837);
#2824=LINE('',#18037,#3838);
#2825=LINE('',#18039,#3839);
#2826=LINE('',#18041,#3840);
#2827=LINE('',#18043,#3841);
#2828=LINE('',#18045,#3842);
#2829=LINE('',#18047,#3843);
#2830=LINE('',#18049,#3844);
#2831=LINE('',#18051,#3845);
#2832=LINE('',#18053,#3846);
#2833=LINE('',#18055,#3847);
#2834=LINE('',#18057,#3848);
#2835=LINE('',#18059,#3849);
#2836=LINE('',#18061,#3850);
#2837=LINE('',#18063,#3851);
#2838=LINE('',#18065,#3852);
#2839=LINE('',#18067,#3853);
#2840=LINE('',#18069,#3854);
#2841=LINE('',#18071,#3855);
#2842=LINE('',#18073,#3856);
#2843=LINE('',#18075,#3857);
#2844=LINE('',#18077,#3858);
#2845=LINE('',#18079,#3859);
#2846=LINE('',#18081,#3860);
#2847=LINE('',#18083,#3861);
#2848=LINE('',#18086,#3862);
#2849=LINE('',#18087,#3863);
#2850=LINE('',#18089,#3864);
#2851=LINE('',#18091,#3865);
#2852=LINE('',#18093,#3866);
#2853=LINE('',#18095,#3867);
#2854=LINE('',#18097,#3868);
#2855=LINE('',#18099,#3869);
#2856=LINE('',#18102,#3870);
#2857=LINE('',#18103,#3871);
#2858=LINE('',#18105,#3872);
#2859=LINE('',#18107,#3873);
#2860=LINE('',#18110,#3874);
#2861=LINE('',#18112,#3875);
#2862=LINE('',#18114,#3876);
#2863=LINE('',#18116,#3877);
#2864=LINE('',#18118,#3878);
#2865=LINE('',#18120,#3879);
#2866=LINE('',#18122,#3880);
#2867=LINE('',#18124,#3881);
#2868=LINE('',#18126,#3882);
#2869=LINE('',#18128,#3883);
#2870=LINE('',#18131,#3884);
#2871=LINE('',#18132,#3885);
#2872=LINE('',#18134,#3886);
#2873=LINE('',#18136,#3887);
#2874=LINE('',#18138,#3888);
#2875=LINE('',#18140,#3889);
#2876=LINE('',#18142,#3890);
#2877=LINE('',#18144,#3891);
#2878=LINE('',#18147,#3892);
#2879=LINE('',#18148,#3893);
#2880=LINE('',#18150,#3894);
#2881=LINE('',#18152,#3895);
#2882=LINE('',#18154,#3896);
#2883=LINE('',#18156,#3897);
#2884=LINE('',#18158,#3898);
#2885=LINE('',#18160,#3899);
#2886=LINE('',#18163,#3900);
#2887=LINE('',#18164,#3901);
#2888=LINE('',#18166,#3902);
#2889=LINE('',#18168,#3903);
#2890=LINE('',#18170,#3904);
#2891=LINE('',#18172,#3905);
#2892=LINE('',#18174,#3906);
#2893=LINE('',#18176,#3907);
#3552=VECTOR('',#13906,1000.);
#3553=VECTOR('',#13909,1000.);
#3554=VECTOR('',#13912,1000.);
#3555=VECTOR('',#13913,1000.);
#3556=VECTOR('',#13914,1000.);
#3557=VECTOR('',#13915,1000.);
#3558=VECTOR('',#13916,1000.);
#3559=VECTOR('',#13919,1000.);
#3560=VECTOR('',#13922,1000.);
#3561=VECTOR('',#13925,1000.);
#3562=VECTOR('',#13928,1000.);
#3563=VECTOR('',#13931,1000.);
#3564=VECTOR('',#13934,1000.);
#3565=VECTOR('',#13937,1000.);
#3566=VECTOR('',#13940,1000.);
#3567=VECTOR('',#13943,1000.);
#3568=VECTOR('',#13946,1000.);
#3569=VECTOR('',#13949,1000.);
#3570=VECTOR('',#13950,1000.);
#3571=VECTOR('',#13951,1000.);
#3572=VECTOR('',#13952,1000.);
#3573=VECTOR('',#13953,1000.);
#3574=VECTOR('',#13954,1000.);
#3575=VECTOR('',#13955,1000.);
#3576=VECTOR('',#13956,1000.);
#3577=VECTOR('',#13959,1000.);
#3578=VECTOR('',#13962,1000.);
#3579=VECTOR('',#13965,1000.);
#3580=VECTOR('',#13968,1000.);
#3581=VECTOR('',#13971,1000.);
#3582=VECTOR('',#13974,1000.);
#3583=VECTOR('',#13977,1000.);
#3584=VECTOR('',#13980,1000.);
#3585=VECTOR('',#13983,1000.);
#3586=VECTOR('',#13986,1000.);
#3587=VECTOR('',#13989,1000.);
#3588=VECTOR('',#13990,1000.);
#3589=VECTOR('',#13991,1000.);
#3590=VECTOR('',#13992,1000.);
#3591=VECTOR('',#13993,1000.);
#3592=VECTOR('',#13994,1000.);
#3593=VECTOR('',#13995,1000.);
#3594=VECTOR('',#13996,1000.);
#3595=VECTOR('',#13999,1000.);
#3596=VECTOR('',#14002,1000.);
#3597=VECTOR('',#14005,1000.);
#3598=VECTOR('',#14008,1000.);
#3599=VECTOR('',#14011,1000.);
#3600=VECTOR('',#14014,1000.);
#3601=VECTOR('',#14017,1000.);
#3602=VECTOR('',#14020,1000.);
#3603=VECTOR('',#14023,1000.);
#3604=VECTOR('',#14026,1000.);
#3605=VECTOR('',#14029,1000.);
#3606=VECTOR('',#14030,1000.);
#3607=VECTOR('',#14031,1000.);
#3608=VECTOR('',#14032,1000.);
#3609=VECTOR('',#14033,1000.);
#3610=VECTOR('',#14034,1000.);
#3611=VECTOR('',#14035,1000.);
#3612=VECTOR('',#14036,1000.);
#3613=VECTOR('',#14039,1000.);
#3614=VECTOR('',#14042,1000.);
#3615=VECTOR('',#14045,1000.);
#3616=VECTOR('',#14048,1000.);
#3617=VECTOR('',#14051,1000.);
#3618=VECTOR('',#14054,1000.);
#3619=VECTOR('',#14057,1000.);
#3620=VECTOR('',#14060,1000.);
#3621=VECTOR('',#14063,1000.);
#3622=VECTOR('',#14066,1000.);
#3623=VECTOR('',#14069,1000.);
#3624=VECTOR('',#14070,1000.);
#3625=VECTOR('',#14071,1000.);
#3626=VECTOR('',#14072,1000.);
#3627=VECTOR('',#14075,1000.);
#3628=VECTOR('',#14078,1000.);
#3629=VECTOR('',#14081,1000.);
#3630=VECTOR('',#14084,1000.);
#3631=VECTOR('',#14087,1000.);
#3632=VECTOR('',#14090,1000.);
#3633=VECTOR('',#14093,1000.);
#3634=VECTOR('',#14096,1000.);
#3635=VECTOR('',#14099,1000.);
#3636=VECTOR('',#14102,1000.);
#3637=VECTOR('',#14103,1000.);
#3638=VECTOR('',#14106,1000.);
#3639=VECTOR('',#14109,1000.);
#3640=VECTOR('',#14112,1000.);
#3641=VECTOR('',#14115,1000.);
#3642=VECTOR('',#14118,1000.);
#3643=VECTOR('',#14121,1000.);
#3644=VECTOR('',#14124,1000.);
#3645=VECTOR('',#14127,1000.);
#3646=VECTOR('',#14130,1000.);
#3647=VECTOR('',#14133,1000.);
#3648=VECTOR('',#14136,1000.);
#3649=VECTOR('',#14139,1000.);
#3650=VECTOR('',#14144,1000.);
#3651=VECTOR('',#14145,1000.);
#3652=VECTOR('',#14146,1000.);
#3653=VECTOR('',#14147,1000.);
#3654=VECTOR('',#14150,1000.);
#3655=VECTOR('',#14153,1000.);
#3656=VECTOR('',#14156,1000.);
#3657=VECTOR('',#14159,1000.);
#3658=VECTOR('',#14162,1000.);
#3659=VECTOR('',#14165,1000.);
#3660=VECTOR('',#14168,1000.);
#3661=VECTOR('',#14171,1000.);
#3662=VECTOR('',#14174,1000.);
#3663=VECTOR('',#14177,1000.);
#3664=VECTOR('',#14180,1000.);
#3665=VECTOR('',#14181,1000.);
#3666=VECTOR('',#14182,1000.);
#3667=VECTOR('',#14183,1000.);
#3668=VECTOR('',#14184,1000.);
#3669=VECTOR('',#14185,1000.);
#3670=VECTOR('',#14186,1000.);
#3671=VECTOR('',#14187,1000.);
#3672=VECTOR('',#14190,1000.);
#3673=VECTOR('',#14193,1000.);
#3674=VECTOR('',#14196,1000.);
#3675=VECTOR('',#14199,1000.);
#3676=VECTOR('',#14202,1000.);
#3677=VECTOR('',#14205,1000.);
#3678=VECTOR('',#14208,1000.);
#3679=VECTOR('',#14211,1000.);
#3680=VECTOR('',#14214,1000.);
#3681=VECTOR('',#14217,1000.);
#3682=VECTOR('',#14220,1000.);
#3683=VECTOR('',#14221,1000.);
#3684=VECTOR('',#14222,1000.);
#3685=VECTOR('',#14223,1000.);
#3686=VECTOR('',#14224,1000.);
#3687=VECTOR('',#14225,1000.);
#3688=VECTOR('',#14226,1000.);
#3689=VECTOR('',#14227,1000.);
#3690=VECTOR('',#14230,1000.);
#3691=VECTOR('',#14233,1000.);
#3692=VECTOR('',#14236,1000.);
#3693=VECTOR('',#14239,1000.);
#3694=VECTOR('',#14242,1000.);
#3695=VECTOR('',#14245,1000.);
#3696=VECTOR('',#14248,1000.);
#3697=VECTOR('',#14251,1000.);
#3698=VECTOR('',#14254,1000.);
#3699=VECTOR('',#14257,1000.);
#3700=VECTOR('',#14260,1000.);
#3701=VECTOR('',#14261,1000.);
#3702=VECTOR('',#14262,1000.);
#3703=VECTOR('',#14263,1000.);
#3704=VECTOR('',#14264,1000.);
#3705=VECTOR('',#14265,1000.);
#3706=VECTOR('',#14266,1000.);
#3707=VECTOR('',#14267,1000.);
#3708=VECTOR('',#14270,1000.);
#3709=VECTOR('',#14273,1000.);
#3710=VECTOR('',#14276,1000.);
#3711=VECTOR('',#14279,1000.);
#3712=VECTOR('',#14282,1000.);
#3713=VECTOR('',#14285,1000.);
#3714=VECTOR('',#14288,1000.);
#3715=VECTOR('',#14291,1000.);
#3716=VECTOR('',#14294,1000.);
#3717=VECTOR('',#14297,1000.);
#3718=VECTOR('',#14300,1000.);
#3719=VECTOR('',#14301,1000.);
#3720=VECTOR('',#14302,1000.);
#3721=VECTOR('',#14303,1000.);
#3722=VECTOR('',#14306,1000.);
#3723=VECTOR('',#14309,1000.);
#3724=VECTOR('',#14312,1000.);
#3725=VECTOR('',#14315,1000.);
#3726=VECTOR('',#14318,1000.);
#3727=VECTOR('',#14321,1000.);
#3728=VECTOR('',#14324,1000.);
#3729=VECTOR('',#14327,1000.);
#3730=VECTOR('',#14330,1000.);
#3731=VECTOR('',#14333,1000.);
#3732=VECTOR('',#14336,1000.);
#3733=VECTOR('',#14339,1000.);
#3734=VECTOR('',#14342,1000.);
#3735=VECTOR('',#14345,1000.);
#3736=VECTOR('',#14348,1000.);
#3737=VECTOR('',#14351,1000.);
#3738=VECTOR('',#14354,1000.);
#3739=VECTOR('',#14357,1000.);
#3740=VECTOR('',#14358,1000.);
#3741=VECTOR('',#14361,1000.);
#3742=VECTOR('',#14364,1000.);
#3743=VECTOR('',#14367,1000.);
#3744=VECTOR('',#14370,1000.);
#3745=VECTOR('',#14373,1000.);
#3746=VECTOR('',#14376,1000.);
#3747=VECTOR('',#14377,1000.);
#3748=VECTOR('',#14380,1000.);
#3749=VECTOR('',#14383,1000.);
#3750=VECTOR('',#14386,1000.);
#3751=VECTOR('',#14389,1000.);
#3752=VECTOR('',#14392,1000.);
#3753=VECTOR('',#14395,1000.);
#3754=VECTOR('',#14398,1000.);
#3755=VECTOR('',#14401,1000.);
#3756=VECTOR('',#14404,1000.);
#3757=VECTOR('',#14407,1000.);
#3758=VECTOR('',#14410,1000.);
#3759=VECTOR('',#14413,1000.);
#3760=VECTOR('',#14416,1000.);
#3761=VECTOR('',#14419,1000.);
#3762=VECTOR('',#14422,1000.);
#3763=VECTOR('',#14425,1000.);
#3764=VECTOR('',#14428,1000.);
#3765=VECTOR('',#14431,1000.);
#3766=VECTOR('',#14434,1000.);
#3767=VECTOR('',#14437,1000.);
#3768=VECTOR('',#14440,1000.);
#3769=VECTOR('',#14443,1000.);
#3770=VECTOR('',#14446,1000.);
#3771=VECTOR('',#14449,1000.);
#3772=VECTOR('',#14452,1000.);
#3773=VECTOR('',#14455,1000.);
#3774=VECTOR('',#14458,1000.);
#3775=VECTOR('',#14461,1000.);
#3776=VECTOR('',#14464,1000.);
#3777=VECTOR('',#14467,1000.);
#3778=VECTOR('',#14470,1000.);
#3779=VECTOR('',#14473,1000.);
#3780=VECTOR('',#14476,1000.);
#3781=VECTOR('',#14479,1000.);
#3782=VECTOR('',#14482,1000.);
#3783=VECTOR('',#14485,1000.);
#3784=VECTOR('',#14488,1000.);
#3785=VECTOR('',#14491,1000.);
#3786=VECTOR('',#14494,1000.);
#3787=VECTOR('',#14497,1000.);
#3788=VECTOR('',#14500,1000.);
#3789=VECTOR('',#14503,1000.);
#3790=VECTOR('',#14506,1000.);
#3791=VECTOR('',#14509,1000.);
#3792=VECTOR('',#14512,1000.);
#3793=VECTOR('',#14515,1000.);
#3794=VECTOR('',#14518,1000.);
#3795=VECTOR('',#14521,1000.);
#3796=VECTOR('',#14524,1000.);
#3797=VECTOR('',#14527,1000.);
#3798=VECTOR('',#14530,1000.);
#3799=VECTOR('',#14533,1000.);
#3800=VECTOR('',#14536,1000.);
#3801=VECTOR('',#14539,1000.);
#3802=VECTOR('',#14542,1000.);
#3803=VECTOR('',#14545,1000.);
#3804=VECTOR('',#14548,1000.);
#3805=VECTOR('',#14551,1000.);
#3806=VECTOR('',#14554,1000.);
#3807=VECTOR('',#14557,1000.);
#3808=VECTOR('',#14560,1000.);
#3809=VECTOR('',#14563,1000.);
#3810=VECTOR('',#14566,1000.);
#3811=VECTOR('',#14569,1000.);
#3812=VECTOR('',#14572,1000.);
#3813=VECTOR('',#14575,1000.);
#3814=VECTOR('',#14578,1000.);
#3815=VECTOR('',#14581,1000.);
#3816=VECTOR('',#14584,1000.);
#3817=VECTOR('',#14587,1000.);
#3818=VECTOR('',#14590,1000.);
#3819=VECTOR('',#14593,1000.);
#3820=VECTOR('',#14596,1000.);
#3821=VECTOR('',#14599,1000.);
#3822=VECTOR('',#14602,1000.);
#3823=VECTOR('',#14605,1000.);
#3824=VECTOR('',#14608,1000.);
#3825=VECTOR('',#14611,1000.);
#3826=VECTOR('',#14614,1000.);
#3827=VECTOR('',#14617,1000.);
#3828=VECTOR('',#14620,1000.);
#3829=VECTOR('',#14623,1000.);
#3830=VECTOR('',#14626,1000.);
#3831=VECTOR('',#14629,1000.);
#3832=VECTOR('',#14632,1000.);
#3833=VECTOR('',#14635,1000.);
#3834=VECTOR('',#14638,1000.);
#3835=VECTOR('',#14641,1000.);
#3836=VECTOR('',#14644,1000.);
#3837=VECTOR('',#14647,1000.);
#3838=VECTOR('',#14650,1000.);
#3839=VECTOR('',#14653,1000.);
#3840=VECTOR('',#14656,1000.);
#3841=VECTOR('',#14659,1000.);
#3842=VECTOR('',#14662,1000.);
#3843=VECTOR('',#14665,1000.);
#3844=VECTOR('',#14668,1000.);
#3845=VECTOR('',#14671,1000.);
#3846=VECTOR('',#14674,1000.);
#3847=VECTOR('',#14677,1000.);
#3848=VECTOR('',#14680,1000.);
#3849=VECTOR('',#14683,1000.);
#3850=VECTOR('',#14686,1000.);
#3851=VECTOR('',#14689,1000.);
#3852=VECTOR('',#14692,1000.);
#3853=VECTOR('',#14695,1000.);
#3854=VECTOR('',#14698,1000.);
#3855=VECTOR('',#14701,1000.);
#3856=VECTOR('',#14704,1000.);
#3857=VECTOR('',#14707,1000.);
#3858=VECTOR('',#14710,1000.);
#3859=VECTOR('',#14713,1000.);
#3860=VECTOR('',#14716,1000.);
#3861=VECTOR('',#14719,1000.);
#3862=VECTOR('',#14724,1000.);
#3863=VECTOR('',#14725,1000.);
#3864=VECTOR('',#14728,1000.);
#3865=VECTOR('',#14731,1000.);
#3866=VECTOR('',#14734,1000.);
#3867=VECTOR('',#14737,1000.);
#3868=VECTOR('',#14740,1000.);
#3869=VECTOR('',#14743,1000.);
#3870=VECTOR('',#14748,1000.);
#3871=VECTOR('',#14749,1000.);
#3872=VECTOR('',#14752,1000.);
#3873=VECTOR('',#14755,1000.);
#3874=VECTOR('',#14760,1000.);
#3875=VECTOR('',#14763,1000.);
#3876=VECTOR('',#14766,1000.);
#3877=VECTOR('',#14769,1000.);
#3878=VECTOR('',#14772,1000.);
#3879=VECTOR('',#14775,1000.);
#3880=VECTOR('',#14778,1000.);
#3881=VECTOR('',#14781,1000.);
#3882=VECTOR('',#14784,1000.);
#3883=VECTOR('',#14787,1000.);
#3884=VECTOR('',#14792,1000.);
#3885=VECTOR('',#14793,1000.);
#3886=VECTOR('',#14796,1000.);
#3887=VECTOR('',#14799,1000.);
#3888=VECTOR('',#14802,1000.);
#3889=VECTOR('',#14805,1000.);
#3890=VECTOR('',#14808,1000.);
#3891=VECTOR('',#14811,1000.);
#3892=VECTOR('',#14816,1000.);
#3893=VECTOR('',#14817,1000.);
#3894=VECTOR('',#14820,1000.);
#3895=VECTOR('',#14823,1000.);
#3896=VECTOR('',#14826,1000.);
#3897=VECTOR('',#14829,1000.);
#3898=VECTOR('',#14832,1000.);
#3899=VECTOR('',#14835,1000.);
#3900=VECTOR('',#14840,1000.);
#3901=VECTOR('',#14841,1000.);
#3902=VECTOR('',#14844,1000.);
#3903=VECTOR('',#14847,1000.);
#3904=VECTOR('',#14850,1000.);
#3905=VECTOR('',#14853,1000.);
#3906=VECTOR('',#14856,1000.);
#3907=VECTOR('',#14859,1000.);
#4312=CIRCLE('',#11714,3.65);
#4313=CIRCLE('',#11715,3.65);
#4314=CIRCLE('',#11717,0.200000403400263);
#4315=CIRCLE('',#11718,0.600000196920858);
#4316=CIRCLE('',#11719,0.200000373597978);
#4317=CIRCLE('',#11720,0.199999419924102);
#4318=CIRCLE('',#11721,0.20000038104856);
#4319=CIRCLE('',#11722,1.99999965375783);
#4320=CIRCLE('',#11723,0.200000284191204);
#4321=CIRCLE('',#11724,0.200000284191204);
#4322=CIRCLE('',#11725,0.200000284191218);
#4323=CIRCLE('',#11726,0.60000037573478);
#4324=CIRCLE('',#11727,0.200000284191204);
#4325=CIRCLE('',#11728,0.20000028419119);
#4326=CIRCLE('',#11729,0.60000037573478);
#4327=CIRCLE('',#11730,0.200000284191218);
#4328=CIRCLE('',#11731,0.200000284191204);
#4329=CIRCLE('',#11732,0.200000284191218);
#4330=CIRCLE('',#11733,1.99999965375781);
#4331=CIRCLE('',#11734,0.200000381048546);
#4332=CIRCLE('',#11735,0.199999419924102);
#4333=CIRCLE('',#11736,0.200000373597978);
#4334=CIRCLE('',#11737,0.600000196920858);
#4335=CIRCLE('',#11738,0.200000403400263);
#4336=CIRCLE('',#11739,0.200000403400263);
#4337=CIRCLE('',#11740,0.600000196920858);
#4338=CIRCLE('',#11741,0.200000373597978);
#4339=CIRCLE('',#11742,0.199999419924102);
#4340=CIRCLE('',#11743,0.200000381048546);
#4341=CIRCLE('',#11744,1.99999965375781);
#4342=CIRCLE('',#11745,0.200000284191204);
#4343=CIRCLE('',#11746,0.200000284191204);
#4344=CIRCLE('',#11747,0.200000284191218);
#4345=CIRCLE('',#11748,0.600000375734794);
#4346=CIRCLE('',#11749,0.200000284191204);
#4347=CIRCLE('',#11750,0.200000284191204);
#4348=CIRCLE('',#11751,0.60000037573478);
#4349=CIRCLE('',#11752,0.200000284191218);
#4350=CIRCLE('',#11753,0.20000028419119);
#4351=CIRCLE('',#11754,0.200000284191218);
#4352=CIRCLE('',#11755,1.9999996537578);
#4353=CIRCLE('',#11756,0.200000381048532);
#4354=CIRCLE('',#11757,0.199999419924102);
#4355=CIRCLE('',#11758,0.200000373597992);
#4356=CIRCLE('',#11759,0.600000196920844);
#4357=CIRCLE('',#11760,0.200000403400263);
#4358=CIRCLE('',#11761,0.999999990441758);
#4359=CIRCLE('',#11762,0.999999990441758);
#4360=CIRCLE('',#11763,0.999999990441772);
#4361=CIRCLE('',#11764,0.999999990441772);
#4362=CIRCLE('',#11765,3.65);
#4363=CIRCLE('',#11766,5.50000000000001);
#4364=CIRCLE('',#11767,3.65);
#4365=CIRCLE('',#11768,5.50000000000001);
#4366=CIRCLE('',#11769,3.65);
#4367=CIRCLE('',#11770,5.50000000000001);
#4368=CIRCLE('',#11771,5.50000000000001);
#4369=CIRCLE('',#11772,0.999999990441758);
#4370=CIRCLE('',#11773,0.999999990441758);
#4371=CIRCLE('',#11774,0.999999990441758);
#4372=CIRCLE('',#11775,0.999999990441758);
#4373=CIRCLE('',#11776,0.999999990441758);
#4374=CIRCLE('',#11777,0.999999990441772);
#4375=CIRCLE('',#11778,0.999999990441772);
#4376=CIRCLE('',#11779,0.999999990441758);
#4377=CIRCLE('',#11780,0.999999990441758);
#4378=CIRCLE('',#11781,0.999999990441758);
#4379=CIRCLE('',#11782,0.999999990441758);
#4380=CIRCLE('',#11783,0.999999990441758);
#4381=CIRCLE('',#11785,0.200000403400263);
#4382=CIRCLE('',#11786,0.600000196920844);
#4383=CIRCLE('',#11787,0.200000373597992);
#4384=CIRCLE('',#11788,0.199999419924102);
#4385=CIRCLE('',#11789,0.200000381048532);
#4386=CIRCLE('',#11790,1.9999996537578);
#4387=CIRCLE('',#11791,0.200000284191218);
#4388=CIRCLE('',#11792,0.20000028419119);
#4389=CIRCLE('',#11793,0.200000284191218);
#4390=CIRCLE('',#11794,0.60000037573478);
#4391=CIRCLE('',#11795,0.200000284191204);
#4392=CIRCLE('',#11796,0.200000284191204);
#4393=CIRCLE('',#11797,0.600000375734794);
#4394=CIRCLE('',#11798,0.200000284191218);
#4395=CIRCLE('',#11799,0.200000284191204);
#4396=CIRCLE('',#11800,0.200000284191204);
#4397=CIRCLE('',#11801,1.99999965375781);
#4398=CIRCLE('',#11802,0.200000381048546);
#4399=CIRCLE('',#11803,0.199999419924102);
#4400=CIRCLE('',#11804,0.200000373597978);
#4401=CIRCLE('',#11805,0.600000196920858);
#4402=CIRCLE('',#11806,0.200000403400263);
#4403=CIRCLE('',#11807,0.200000403400263);
#4404=CIRCLE('',#11808,0.600000196920858);
#4405=CIRCLE('',#11809,0.200000373597978);
#4406=CIRCLE('',#11810,0.199999419924102);
#4407=CIRCLE('',#11811,0.200000381048546);
#4408=CIRCLE('',#11812,1.99999965375781);
#4409=CIRCLE('',#11813,0.200000284191218);
#4410=CIRCLE('',#11814,0.200000284191204);
#4411=CIRCLE('',#11815,0.200000284191218);
#4412=CIRCLE('',#11816,0.60000037573478);
#4413=CIRCLE('',#11817,0.20000028419119);
#4414=CIRCLE('',#11818,0.200000284191204);
#4415=CIRCLE('',#11819,0.60000037573478);
#4416=CIRCLE('',#11820,0.200000284191218);
#4417=CIRCLE('',#11821,0.200000284191204);
#4418=CIRCLE('',#11822,0.200000284191204);
#4419=CIRCLE('',#11823,1.99999965375783);
#4420=CIRCLE('',#11824,0.20000038104856);
#4421=CIRCLE('',#11825,0.199999419924102);
#4422=CIRCLE('',#11826,0.200000373597978);
#4423=CIRCLE('',#11827,0.600000196920858);
#4424=CIRCLE('',#11828,0.200000403400263);
#4425=CIRCLE('',#11829,0.999999990441758);
#4426=CIRCLE('',#11830,0.999999990441772);
#4427=CIRCLE('',#11831,0.999999990441772);
#4428=CIRCLE('',#11832,0.999999990441758);
#4429=CIRCLE('',#11833,0.999999990441758);
#4430=CIRCLE('',#11834,0.999999990441758);
#4431=CIRCLE('',#11835,0.999999990441758);
#4432=CIRCLE('',#11836,0.999999990441758);
#4433=CIRCLE('',#11837,0.999999990441758);
#4434=CIRCLE('',#11838,0.999999990441758);
#4435=CIRCLE('',#11839,0.999999990441758);
#4436=CIRCLE('',#11840,0.999999990441758);
#4437=CIRCLE('',#11841,0.999999990441758);
#4438=CIRCLE('',#11842,0.999999990441758);
#4439=CIRCLE('',#11843,0.999999990441772);
#4440=CIRCLE('',#11844,0.999999990441772);
#4441=CIRCLE('',#11845,3.65);
#4442=CIRCLE('',#11846,5.50000000000001);
#4443=CIRCLE('',#11847,5.50000000000001);
#4444=CIRCLE('',#11848,3.65);
#4445=CIRCLE('',#11849,5.50000000000001);
#4446=CIRCLE('',#11850,3.65);
#4447=CIRCLE('',#11851,5.50000000000001);
#5060=VERTEX_POINT('',#17193);
#5061=VERTEX_POINT('',#17194);
#5062=VERTEX_POINT('',#17196);
#5063=VERTEX_POINT('',#17198);
#5064=VERTEX_POINT('',#17202);
#5065=VERTEX_POINT('',#17203);
#5066=VERTEX_POINT('',#17205);
#5067=VERTEX_POINT('',#17207);
#5068=VERTEX_POINT('',#17209);
#5069=VERTEX_POINT('',#17211);
#5070=VERTEX_POINT('',#17213);
#5071=VERTEX_POINT('',#17215);
#5072=VERTEX_POINT('',#17217);
#5073=VERTEX_POINT('',#17219);
#5074=VERTEX_POINT('',#17221);
#5075=VERTEX_POINT('',#17223);
#5076=VERTEX_POINT('',#17225);
#5077=VERTEX_POINT('',#17227);
#5078=VERTEX_POINT('',#17229);
#5079=VERTEX_POINT('',#17231);
#5080=VERTEX_POINT('',#17233);
#5081=VERTEX_POINT('',#17235);
#5082=VERTEX_POINT('',#17237);
#5083=VERTEX_POINT('',#17239);
#5084=VERTEX_POINT('',#17241);
#5085=VERTEX_POINT('',#17243);
#5086=VERTEX_POINT('',#17245);
#5087=VERTEX_POINT('',#17247);
#5088=VERTEX_POINT('',#17249);
#5089=VERTEX_POINT('',#17251);
#5090=VERTEX_POINT('',#17253);
#5091=VERTEX_POINT('',#17255);
#5092=VERTEX_POINT('',#17257);
#5093=VERTEX_POINT('',#17259);
#5094=VERTEX_POINT('',#17261);
#5095=VERTEX_POINT('',#17263);
#5096=VERTEX_POINT('',#17265);
#5097=VERTEX_POINT('',#17267);
#5098=VERTEX_POINT('',#17269);
#5099=VERTEX_POINT('',#17271);
#5100=VERTEX_POINT('',#17273);
#5101=VERTEX_POINT('',#17275);
#5102=VERTEX_POINT('',#17277);
#5103=VERTEX_POINT('',#17279);
#5104=VERTEX_POINT('',#17281);
#5105=VERTEX_POINT('',#17283);
#5106=VERTEX_POINT('',#17285);
#5107=VERTEX_POINT('',#17287);
#5108=VERTEX_POINT('',#17289);
#5109=VERTEX_POINT('',#17291);
#5110=VERTEX_POINT('',#17293);
#5111=VERTEX_POINT('',#17295);
#5112=VERTEX_POINT('',#17297);
#5113=VERTEX_POINT('',#17299);
#5114=VERTEX_POINT('',#17301);
#5115=VERTEX_POINT('',#17303);
#5116=VERTEX_POINT('',#17305);
#5117=VERTEX_POINT('',#17307);
#5118=VERTEX_POINT('',#17309);
#5119=VERTEX_POINT('',#17311);
#5120=VERTEX_POINT('',#17313);
#5121=VERTEX_POINT('',#17315);
#5122=VERTEX_POINT('',#17317);
#5123=VERTEX_POINT('',#17319);
#5124=VERTEX_POINT('',#17321);
#5125=VERTEX_POINT('',#17323);
#5126=VERTEX_POINT('',#17325);
#5127=VERTEX_POINT('',#17327);
#5128=VERTEX_POINT('',#17329);
#5129=VERTEX_POINT('',#17331);
#5130=VERTEX_POINT('',#17333);
#5131=VERTEX_POINT('',#17335);
#5132=VERTEX_POINT('',#17337);
#5133=VERTEX_POINT('',#17339);
#5134=VERTEX_POINT('',#17341);
#5135=VERTEX_POINT('',#17343);
#5136=VERTEX_POINT('',#17345);
#5137=VERTEX_POINT('',#17347);
#5138=VERTEX_POINT('',#17349);
#5139=VERTEX_POINT('',#17351);
#5140=VERTEX_POINT('',#17353);
#5141=VERTEX_POINT('',#17355);
#5142=VERTEX_POINT('',#17357);
#5143=VERTEX_POINT('',#17359);
#5144=VERTEX_POINT('',#17361);
#5145=VERTEX_POINT('',#17363);
#5146=VERTEX_POINT('',#17365);
#5147=VERTEX_POINT('',#17367);
#5148=VERTEX_POINT('',#17369);
#5149=VERTEX_POINT('',#17371);
#5150=VERTEX_POINT('',#17373);
#5151=VERTEX_POINT('',#17375);
#5152=VERTEX_POINT('',#17377);
#5153=VERTEX_POINT('',#17379);
#5154=VERTEX_POINT('',#17381);
#5155=VERTEX_POINT('',#17383);
#5156=VERTEX_POINT('',#17385);
#5157=VERTEX_POINT('',#17387);
#5158=VERTEX_POINT('',#17389);
#5159=VERTEX_POINT('',#17391);
#5160=VERTEX_POINT('',#17393);
#5161=VERTEX_POINT('',#17395);
#5162=VERTEX_POINT('',#17397);
#5163=VERTEX_POINT('',#17399);
#5164=VERTEX_POINT('',#17401);
#5165=VERTEX_POINT('',#17403);
#5166=VERTEX_POINT('',#17405);
#5167=VERTEX_POINT('',#17407);
#5168=VERTEX_POINT('',#17409);
#5169=VERTEX_POINT('',#17411);
#5170=VERTEX_POINT('',#17413);
#5171=VERTEX_POINT('',#17415);
#5172=VERTEX_POINT('',#17417);
#5173=VERTEX_POINT('',#17419);
#5174=VERTEX_POINT('',#17421);
#5175=VERTEX_POINT('',#17423);
#5176=VERTEX_POINT('',#17425);
#5177=VERTEX_POINT('',#17427);
#5178=VERTEX_POINT('',#17429);
#5179=VERTEX_POINT('',#17431);
#5180=VERTEX_POINT('',#17434);
#5181=VERTEX_POINT('',#17435);
#5182=VERTEX_POINT('',#17437);
#5183=VERTEX_POINT('',#17439);
#5184=VERTEX_POINT('',#17441);
#5185=VERTEX_POINT('',#17443);
#5186=VERTEX_POINT('',#17445);
#5187=VERTEX_POINT('',#17447);
#5188=VERTEX_POINT('',#17450);
#5189=VERTEX_POINT('',#17451);
#5190=VERTEX_POINT('',#17453);
#5191=VERTEX_POINT('',#17455);
#5192=VERTEX_POINT('',#17457);
#5193=VERTEX_POINT('',#17459);
#5194=VERTEX_POINT('',#17461);
#5195=VERTEX_POINT('',#17463);
#5196=VERTEX_POINT('',#17465);
#5197=VERTEX_POINT('',#17467);
#5198=VERTEX_POINT('',#17469);
#5199=VERTEX_POINT('',#17471);
#5200=VERTEX_POINT('',#17473);
#5201=VERTEX_POINT('',#17476);
#5202=VERTEX_POINT('',#17479);
#5203=VERTEX_POINT('',#17480);
#5204=VERTEX_POINT('',#17482);
#5205=VERTEX_POINT('',#17484);
#5206=VERTEX_POINT('',#17486);
#5207=VERTEX_POINT('',#17488);
#5208=VERTEX_POINT('',#17490);
#5209=VERTEX_POINT('',#17492);
#5210=VERTEX_POINT('',#17495);
#5211=VERTEX_POINT('',#17496);
#5212=VERTEX_POINT('',#17498);
#5213=VERTEX_POINT('',#17500);
#5214=VERTEX_POINT('',#17502);
#5215=VERTEX_POINT('',#17504);
#5216=VERTEX_POINT('',#17506);
#5217=VERTEX_POINT('',#17508);
#5218=VERTEX_POINT('',#17511);
#5219=VERTEX_POINT('',#17512);
#5220=VERTEX_POINT('',#17514);
#5221=VERTEX_POINT('',#17516);
#5222=VERTEX_POINT('',#17518);
#5223=VERTEX_POINT('',#17520);
#5224=VERTEX_POINT('',#17522);
#5225=VERTEX_POINT('',#17524);
#5226=VERTEX_POINT('',#17528);
#5227=VERTEX_POINT('',#17529);
#5228=VERTEX_POINT('',#17531);
#5229=VERTEX_POINT('',#17533);
#5230=VERTEX_POINT('',#17535);
#5231=VERTEX_POINT('',#17537);
#5232=VERTEX_POINT('',#17539);
#5233=VERTEX_POINT('',#17541);
#5234=VERTEX_POINT('',#17543);
#5235=VERTEX_POINT('',#17545);
#5236=VERTEX_POINT('',#17547);
#5237=VERTEX_POINT('',#17549);
#5238=VERTEX_POINT('',#17551);
#5239=VERTEX_POINT('',#17553);
#5240=VERTEX_POINT('',#17555);
#5241=VERTEX_POINT('',#17557);
#5242=VERTEX_POINT('',#17559);
#5243=VERTEX_POINT('',#17561);
#5244=VERTEX_POINT('',#17563);
#5245=VERTEX_POINT('',#17565);
#5246=VERTEX_POINT('',#17567);
#5247=VERTEX_POINT('',#17569);
#5248=VERTEX_POINT('',#17571);
#5249=VERTEX_POINT('',#17573);
#5250=VERTEX_POINT('',#17575);
#5251=VERTEX_POINT('',#17577);
#5252=VERTEX_POINT('',#17579);
#5253=VERTEX_POINT('',#17581);
#5254=VERTEX_POINT('',#17583);
#5255=VERTEX_POINT('',#17585);
#5256=VERTEX_POINT('',#17587);
#5257=VERTEX_POINT('',#17589);
#5258=VERTEX_POINT('',#17591);
#5259=VERTEX_POINT('',#17593);
#5260=VERTEX_POINT('',#17595);
#5261=VERTEX_POINT('',#17597);
#5262=VERTEX_POINT('',#17599);
#5263=VERTEX_POINT('',#17601);
#5264=VERTEX_POINT('',#17603);
#5265=VERTEX_POINT('',#17605);
#5266=VERTEX_POINT('',#17607);
#5267=VERTEX_POINT('',#17609);
#5268=VERTEX_POINT('',#17611);
#5269=VERTEX_POINT('',#17613);
#5270=VERTEX_POINT('',#17615);
#5271=VERTEX_POINT('',#17617);
#5272=VERTEX_POINT('',#17619);
#5273=VERTEX_POINT('',#17621);
#5274=VERTEX_POINT('',#17623);
#5275=VERTEX_POINT('',#17625);
#5276=VERTEX_POINT('',#17627);
#5277=VERTEX_POINT('',#17629);
#5278=VERTEX_POINT('',#17631);
#5279=VERTEX_POINT('',#17633);
#5280=VERTEX_POINT('',#17635);
#5281=VERTEX_POINT('',#17637);
#5282=VERTEX_POINT('',#17639);
#5283=VERTEX_POINT('',#17641);
#5284=VERTEX_POINT('',#17643);
#5285=VERTEX_POINT('',#17645);
#5286=VERTEX_POINT('',#17647);
#5287=VERTEX_POINT('',#17649);
#5288=VERTEX_POINT('',#17651);
#5289=VERTEX_POINT('',#17653);
#5290=VERTEX_POINT('',#17655);
#5291=VERTEX_POINT('',#17657);
#5292=VERTEX_POINT('',#17659);
#5293=VERTEX_POINT('',#17661);
#5294=VERTEX_POINT('',#17663);
#5295=VERTEX_POINT('',#17665);
#5296=VERTEX_POINT('',#17667);
#5297=VERTEX_POINT('',#17669);
#5298=VERTEX_POINT('',#17671);
#5299=VERTEX_POINT('',#17673);
#5300=VERTEX_POINT('',#17675);
#5301=VERTEX_POINT('',#17677);
#5302=VERTEX_POINT('',#17679);
#5303=VERTEX_POINT('',#17681);
#5304=VERTEX_POINT('',#17683);
#5305=VERTEX_POINT('',#17685);
#5306=VERTEX_POINT('',#17687);
#5307=VERTEX_POINT('',#17689);
#5308=VERTEX_POINT('',#17691);
#5309=VERTEX_POINT('',#17693);
#5310=VERTEX_POINT('',#17695);
#5311=VERTEX_POINT('',#17697);
#5312=VERTEX_POINT('',#17699);
#5313=VERTEX_POINT('',#17701);
#5314=VERTEX_POINT('',#17703);
#5315=VERTEX_POINT('',#17705);
#5316=VERTEX_POINT('',#17707);
#5317=VERTEX_POINT('',#17709);
#5318=VERTEX_POINT('',#17711);
#5319=VERTEX_POINT('',#17713);
#5320=VERTEX_POINT('',#17715);
#5321=VERTEX_POINT('',#17717);
#5322=VERTEX_POINT('',#17719);
#5323=VERTEX_POINT('',#17721);
#5324=VERTEX_POINT('',#17723);
#5325=VERTEX_POINT('',#17725);
#5326=VERTEX_POINT('',#17727);
#5327=VERTEX_POINT('',#17729);
#5328=VERTEX_POINT('',#17731);
#5329=VERTEX_POINT('',#17733);
#5330=VERTEX_POINT('',#17735);
#5331=VERTEX_POINT('',#17737);
#5332=VERTEX_POINT('',#17739);
#5333=VERTEX_POINT('',#17741);
#5334=VERTEX_POINT('',#17743);
#5335=VERTEX_POINT('',#17745);
#5336=VERTEX_POINT('',#17747);
#5337=VERTEX_POINT('',#17749);
#5338=VERTEX_POINT('',#17751);
#5339=VERTEX_POINT('',#17753);
#5340=VERTEX_POINT('',#17755);
#5341=VERTEX_POINT('',#17757);
#5342=VERTEX_POINT('',#17760);
#5343=VERTEX_POINT('',#17761);
#5344=VERTEX_POINT('',#17763);
#5345=VERTEX_POINT('',#17765);
#5346=VERTEX_POINT('',#17767);
#5347=VERTEX_POINT('',#17769);
#5348=VERTEX_POINT('',#17771);
#5349=VERTEX_POINT('',#17773);
#5350=VERTEX_POINT('',#17776);
#5351=VERTEX_POINT('',#17777);
#5352=VERTEX_POINT('',#17779);
#5353=VERTEX_POINT('',#17781);
#5354=VERTEX_POINT('',#17783);
#5355=VERTEX_POINT('',#17785);
#5356=VERTEX_POINT('',#17787);
#5357=VERTEX_POINT('',#17789);
#5358=VERTEX_POINT('',#17792);
#5359=VERTEX_POINT('',#17793);
#5360=VERTEX_POINT('',#17795);
#5361=VERTEX_POINT('',#17797);
#5362=VERTEX_POINT('',#17799);
#5363=VERTEX_POINT('',#17801);
#5364=VERTEX_POINT('',#17803);
#5365=VERTEX_POINT('',#17805);
#5366=VERTEX_POINT('',#17808);
#5367=VERTEX_POINT('',#17809);
#5368=VERTEX_POINT('',#17811);
#5369=VERTEX_POINT('',#17813);
#5370=VERTEX_POINT('',#17815);
#5371=VERTEX_POINT('',#17817);
#5372=VERTEX_POINT('',#17819);
#5373=VERTEX_POINT('',#17821);
#5374=VERTEX_POINT('',#17824);
#5375=VERTEX_POINT('',#17825);
#5376=VERTEX_POINT('',#17827);
#5377=VERTEX_POINT('',#17829);
#5378=VERTEX_POINT('',#17832);
#5379=VERTEX_POINT('',#17834);
#5380=VERTEX_POINT('',#17836);
#5381=VERTEX_POINT('',#17838);
#5382=VERTEX_POINT('',#17840);
#5383=VERTEX_POINT('',#17842);
#5384=VERTEX_POINT('',#17844);
#5385=VERTEX_POINT('',#17846);
#5386=VERTEX_POINT('',#17848);
#5387=VERTEX_POINT('',#17850);
#6323=EDGE_CURVE('',#5060,#5061,#4312,.T.);
#6324=EDGE_CURVE('',#5061,#5062,#2538,.T.);
#6325=EDGE_CURVE('',#5063,#5062,#4313,.T.);
#6326=EDGE_CURVE('',#5060,#5063,#2539,.T.);
#6327=EDGE_CURVE('',#5064,#5065,#2540,.T.);
#6328=EDGE_CURVE('',#5065,#5066,#2541,.T.);
#6329=EDGE_CURVE('',#5066,#5067,#2542,.T.);
#6330=EDGE_CURVE('',#5067,#5068,#2543,.T.);
#6331=EDGE_CURVE('',#5068,#5069,#2544,.T.);
#6332=EDGE_CURVE('',#5069,#5070,#4314,.T.);
#6333=EDGE_CURVE('',#5070,#5071,#2545,.T.);
#6334=EDGE_CURVE('',#5071,#5072,#4315,.T.);
#6335=EDGE_CURVE('',#5072,#5073,#2546,.T.);
#6336=EDGE_CURVE('',#5073,#5074,#4316,.T.);
#6337=EDGE_CURVE('',#5074,#5075,#2547,.T.);
#6338=EDGE_CURVE('',#5075,#5076,#4317,.T.);
#6339=EDGE_CURVE('',#5076,#5077,#2548,.T.);
#6340=EDGE_CURVE('',#5077,#5078,#4318,.T.);
#6341=EDGE_CURVE('',#5078,#5079,#2549,.T.);
#6342=EDGE_CURVE('',#5079,#5080,#4319,.T.);
#6343=EDGE_CURVE('',#5080,#5081,#2550,.T.);
#6344=EDGE_CURVE('',#5081,#5082,#4320,.T.);
#6345=EDGE_CURVE('',#5082,#5083,#2551,.T.);
#6346=EDGE_CURVE('',#5083,#5084,#4321,.T.);
#6347=EDGE_CURVE('',#5084,#5085,#2552,.T.);
#6348=EDGE_CURVE('',#5085,#5086,#4322,.T.);
#6349=EDGE_CURVE('',#5086,#5087,#2553,.T.);
#6350=EDGE_CURVE('',#5087,#5088,#4323,.T.);
#6351=EDGE_CURVE('',#5088,#5089,#2554,.T.);
#6352=EDGE_CURVE('',#5089,#5090,#4324,.T.);
#6353=EDGE_CURVE('',#5090,#5091,#2555,.T.);
#6354=EDGE_CURVE('',#5091,#5092,#2556,.T.);
#6355=EDGE_CURVE('',#5092,#5093,#2557,.T.);
#6356=EDGE_CURVE('',#5093,#5094,#2558,.T.);
#6357=EDGE_CURVE('',#5094,#5095,#2559,.T.);
#6358=EDGE_CURVE('',#5095,#5096,#2560,.T.);
#6359=EDGE_CURVE('',#5096,#5097,#2561,.T.);
#6360=EDGE_CURVE('',#5097,#5098,#2562,.T.);
#6361=EDGE_CURVE('',#5098,#5099,#4325,.T.);
#6362=EDGE_CURVE('',#5099,#5100,#2563,.T.);
#6363=EDGE_CURVE('',#5100,#5101,#4326,.T.);
#6364=EDGE_CURVE('',#5101,#5102,#2564,.T.);
#6365=EDGE_CURVE('',#5102,#5103,#4327,.T.);
#6366=EDGE_CURVE('',#5103,#5104,#2565,.T.);
#6367=EDGE_CURVE('',#5104,#5105,#4328,.T.);
#6368=EDGE_CURVE('',#5105,#5106,#2566,.T.);
#6369=EDGE_CURVE('',#5106,#5107,#4329,.T.);
#6370=EDGE_CURVE('',#5107,#5108,#2567,.T.);
#6371=EDGE_CURVE('',#5108,#5109,#4330,.T.);
#6372=EDGE_CURVE('',#5109,#5110,#2568,.T.);
#6373=EDGE_CURVE('',#5110,#5111,#4331,.T.);
#6374=EDGE_CURVE('',#5111,#5112,#2569,.T.);
#6375=EDGE_CURVE('',#5112,#5113,#4332,.T.);
#6376=EDGE_CURVE('',#5113,#5114,#2570,.T.);
#6377=EDGE_CURVE('',#5114,#5115,#4333,.T.);
#6378=EDGE_CURVE('',#5115,#5116,#2571,.T.);
#6379=EDGE_CURVE('',#5116,#5117,#4334,.T.);
#6380=EDGE_CURVE('',#5117,#5118,#2572,.T.);
#6381=EDGE_CURVE('',#5118,#5119,#4335,.T.);
#6382=EDGE_CURVE('',#5119,#5120,#2573,.T.);
#6383=EDGE_CURVE('',#5120,#5121,#2574,.T.);
#6384=EDGE_CURVE('',#5121,#5122,#2575,.T.);
#6385=EDGE_CURVE('',#5122,#5123,#2576,.T.);
#6386=EDGE_CURVE('',#5123,#5124,#2577,.T.);
#6387=EDGE_CURVE('',#5124,#5125,#2578,.T.);
#6388=EDGE_CURVE('',#5125,#5126,#2579,.T.);
#6389=EDGE_CURVE('',#5126,#5127,#2580,.T.);
#6390=EDGE_CURVE('',#5127,#5128,#4336,.T.);
#6391=EDGE_CURVE('',#5128,#5129,#2581,.T.);
#6392=EDGE_CURVE('',#5129,#5130,#4337,.T.);
#6393=EDGE_CURVE('',#5130,#5131,#2582,.T.);
#6394=EDGE_CURVE('',#5131,#5132,#4338,.T.);
#6395=EDGE_CURVE('',#5132,#5133,#2583,.T.);
#6396=EDGE_CURVE('',#5133,#5134,#4339,.T.);
#6397=EDGE_CURVE('',#5134,#5135,#2584,.T.);
#6398=EDGE_CURVE('',#5135,#5136,#4340,.T.);
#6399=EDGE_CURVE('',#5136,#5137,#2585,.T.);
#6400=EDGE_CURVE('',#5137,#5138,#4341,.T.);
#6401=EDGE_CURVE('',#5138,#5139,#2586,.T.);
#6402=EDGE_CURVE('',#5139,#5140,#4342,.T.);
#6403=EDGE_CURVE('',#5140,#5141,#2587,.T.);
#6404=EDGE_CURVE('',#5141,#5142,#4343,.T.);
#6405=EDGE_CURVE('',#5142,#5143,#2588,.T.);
#6406=EDGE_CURVE('',#5143,#5144,#4344,.T.);
#6407=EDGE_CURVE('',#5144,#5145,#2589,.T.);
#6408=EDGE_CURVE('',#5145,#5146,#4345,.T.);
#6409=EDGE_CURVE('',#5146,#5147,#2590,.T.);
#6410=EDGE_CURVE('',#5147,#5148,#4346,.T.);
#6411=EDGE_CURVE('',#5148,#5149,#2591,.T.);
#6412=EDGE_CURVE('',#5149,#5150,#2592,.T.);
#6413=EDGE_CURVE('',#5150,#5151,#2593,.T.);
#6414=EDGE_CURVE('',#5151,#5152,#2594,.T.);
#6415=EDGE_CURVE('',#5152,#5153,#2595,.T.);
#6416=EDGE_CURVE('',#5153,#5154,#2596,.T.);
#6417=EDGE_CURVE('',#5154,#5155,#2597,.T.);
#6418=EDGE_CURVE('',#5155,#5156,#2598,.T.);
#6419=EDGE_CURVE('',#5156,#5157,#4347,.T.);
#6420=EDGE_CURVE('',#5157,#5158,#2599,.T.);
#6421=EDGE_CURVE('',#5158,#5159,#4348,.T.);
#6422=EDGE_CURVE('',#5159,#5160,#2600,.T.);
#6423=EDGE_CURVE('',#5160,#5161,#4349,.T.);
#6424=EDGE_CURVE('',#5161,#5162,#2601,.T.);
#6425=EDGE_CURVE('',#5162,#5163,#4350,.T.);
#6426=EDGE_CURVE('',#5163,#5164,#2602,.T.);
#6427=EDGE_CURVE('',#5164,#5165,#4351,.T.);
#6428=EDGE_CURVE('',#5165,#5166,#2603,.T.);
#6429=EDGE_CURVE('',#5166,#5167,#4352,.T.);
#6430=EDGE_CURVE('',#5167,#5168,#2604,.T.);
#6431=EDGE_CURVE('',#5168,#5169,#4353,.T.);
#6432=EDGE_CURVE('',#5169,#5170,#2605,.T.);
#6433=EDGE_CURVE('',#5170,#5171,#4354,.T.);
#6434=EDGE_CURVE('',#5171,#5172,#2606,.T.);
#6435=EDGE_CURVE('',#5172,#5173,#4355,.T.);
#6436=EDGE_CURVE('',#5173,#5174,#2607,.T.);
#6437=EDGE_CURVE('',#5174,#5175,#4356,.T.);
#6438=EDGE_CURVE('',#5175,#5176,#2608,.T.);
#6439=EDGE_CURVE('',#5176,#5177,#4357,.T.);
#6440=EDGE_CURVE('',#5177,#5178,#2609,.T.);
#6441=EDGE_CURVE('',#5178,#5179,#2610,.T.);
#6442=EDGE_CURVE('',#5179,#5064,#2611,.T.);
#6443=EDGE_CURVE('',#5180,#5181,#2612,.T.);
#6444=EDGE_CURVE('',#5182,#5180,#4358,.T.);
#6445=EDGE_CURVE('',#5183,#5182,#2613,.T.);
#6446=EDGE_CURVE('',#5184,#5183,#4359,.T.);
#6447=EDGE_CURVE('',#5185,#5184,#2614,.T.);
#6448=EDGE_CURVE('',#5186,#5185,#4360,.T.);
#6449=EDGE_CURVE('',#5187,#5186,#2615,.T.);
#6450=EDGE_CURVE('',#5181,#5187,#4361,.T.);
#6451=EDGE_CURVE('',#5188,#5189,#2616,.T.);
#6452=EDGE_CURVE('',#5190,#5188,#4362,.T.);
#6453=EDGE_CURVE('',#5191,#5190,#2617,.T.);
#6454=EDGE_CURVE('',#5192,#5191,#4363,.T.);
#6455=EDGE_CURVE('',#5193,#5192,#2618,.T.);
#6456=EDGE_CURVE('',#5194,#5193,#4364,.T.);
#6457=EDGE_CURVE('',#5195,#5194,#2619,.T.);
#6458=EDGE_CURVE('',#5196,#5195,#4365,.T.);
#6459=EDGE_CURVE('',#5197,#5196,#2620,.T.);
#6460=EDGE_CURVE('',#5198,#5197,#4366,.T.);
#6461=EDGE_CURVE('',#5199,#5198,#2621,.T.);
#6462=EDGE_CURVE('',#5200,#5199,#4367,.T.);
#6463=EDGE_CURVE('',#5061,#5200,#2622,.T.);
#6464=EDGE_CURVE('',#5201,#5060,#2623,.T.);
#6465=EDGE_CURVE('',#5189,#5201,#4368,.T.);
#6466=EDGE_CURVE('',#5202,#5203,#2624,.T.);
#6467=EDGE_CURVE('',#5204,#5202,#4369,.T.);
#6468=EDGE_CURVE('',#5205,#5204,#2625,.T.);
#6469=EDGE_CURVE('',#5206,#5205,#4370,.T.);
#6470=EDGE_CURVE('',#5207,#5206,#2626,.T.);
#6471=EDGE_CURVE('',#5208,#5207,#4371,.T.);
#6472=EDGE_CURVE('',#5209,#5208,#2627,.T.);
#6473=EDGE_CURVE('',#5203,#5209,#4372,.T.);
#6474=EDGE_CURVE('',#5210,#5211,#2628,.T.);
#6475=EDGE_CURVE('',#5212,#5210,#4373,.T.);
#6476=EDGE_CURVE('',#5213,#5212,#2629,.T.);
#6477=EDGE_CURVE('',#5214,#5213,#4374,.T.);
#6478=EDGE_CURVE('',#5215,#5214,#2630,.T.);
#6479=EDGE_CURVE('',#5216,#5215,#4375,.T.);
#6480=EDGE_CURVE('',#5217,#5216,#2631,.T.);
#6481=EDGE_CURVE('',#5211,#5217,#4376,.T.);
#6482=EDGE_CURVE('',#5218,#5219,#2632,.T.);
#6483=EDGE_CURVE('',#5220,#5218,#4377,.T.);
#6484=EDGE_CURVE('',#5221,#5220,#2633,.T.);
#6485=EDGE_CURVE('',#5222,#5221,#4378,.T.);
#6486=EDGE_CURVE('',#5223,#5222,#2634,.T.);
#6487=EDGE_CURVE('',#5224,#5223,#4379,.T.);
#6488=EDGE_CURVE('',#5225,#5224,#2635,.T.);
#6489=EDGE_CURVE('',#5219,#5225,#4380,.T.);
#6490=EDGE_CURVE('',#5226,#5227,#2636,.T.);
#6491=EDGE_CURVE('',#5228,#5226,#2637,.T.);
#6492=EDGE_CURVE('',#5229,#5228,#2638,.T.);
#6493=EDGE_CURVE('',#5230,#5229,#2639,.T.);
#6494=EDGE_CURVE('',#5231,#5230,#4381,.T.);
#6495=EDGE_CURVE('',#5232,#5231,#2640,.T.);
#6496=EDGE_CURVE('',#5233,#5232,#4382,.T.);
#6497=EDGE_CURVE('',#5234,#5233,#2641,.T.);
#6498=EDGE_CURVE('',#5235,#5234,#4383,.T.);
#6499=EDGE_CURVE('',#5236,#5235,#2642,.T.);
#6500=EDGE_CURVE('',#5237,#5236,#4384,.T.);
#6501=EDGE_CURVE('',#5238,#5237,#2643,.T.);
#6502=EDGE_CURVE('',#5239,#5238,#4385,.T.);
#6503=EDGE_CURVE('',#5240,#5239,#2644,.T.);
#6504=EDGE_CURVE('',#5241,#5240,#4386,.T.);
#6505=EDGE_CURVE('',#5242,#5241,#2645,.T.);
#6506=EDGE_CURVE('',#5243,#5242,#4387,.T.);
#6507=EDGE_CURVE('',#5244,#5243,#2646,.T.);
#6508=EDGE_CURVE('',#5245,#5244,#4388,.T.);
#6509=EDGE_CURVE('',#5246,#5245,#2647,.T.);
#6510=EDGE_CURVE('',#5247,#5246,#4389,.T.);
#6511=EDGE_CURVE('',#5248,#5247,#2648,.T.);
#6512=EDGE_CURVE('',#5249,#5248,#4390,.T.);
#6513=EDGE_CURVE('',#5250,#5249,#2649,.T.);
#6514=EDGE_CURVE('',#5251,#5250,#4391,.T.);
#6515=EDGE_CURVE('',#5252,#5251,#2650,.T.);
#6516=EDGE_CURVE('',#5253,#5252,#2651,.T.);
#6517=EDGE_CURVE('',#5254,#5253,#2652,.T.);
#6518=EDGE_CURVE('',#5255,#5254,#2653,.T.);
#6519=EDGE_CURVE('',#5256,#5255,#2654,.T.);
#6520=EDGE_CURVE('',#5257,#5256,#2655,.T.);
#6521=EDGE_CURVE('',#5258,#5257,#2656,.T.);
#6522=EDGE_CURVE('',#5259,#5258,#2657,.T.);
#6523=EDGE_CURVE('',#5260,#5259,#4392,.T.);
#6524=EDGE_CURVE('',#5261,#5260,#2658,.T.);
#6525=EDGE_CURVE('',#5262,#5261,#4393,.T.);
#6526=EDGE_CURVE('',#5263,#5262,#2659,.T.);
#6527=EDGE_CURVE('',#5264,#5263,#4394,.T.);
#6528=EDGE_CURVE('',#5265,#5264,#2660,.T.);
#6529=EDGE_CURVE('',#5266,#5265,#4395,.T.);
#6530=EDGE_CURVE('',#5267,#5266,#2661,.T.);
#6531=EDGE_CURVE('',#5268,#5267,#4396,.T.);
#6532=EDGE_CURVE('',#5269,#5268,#2662,.T.);
#6533=EDGE_CURVE('',#5270,#5269,#4397,.T.);
#6534=EDGE_CURVE('',#5271,#5270,#2663,.T.);
#6535=EDGE_CURVE('',#5272,#5271,#4398,.T.);
#6536=EDGE_CURVE('',#5273,#5272,#2664,.T.);
#6537=EDGE_CURVE('',#5274,#5273,#4399,.T.);
#6538=EDGE_CURVE('',#5275,#5274,#2665,.T.);
#6539=EDGE_CURVE('',#5276,#5275,#4400,.T.);
#6540=EDGE_CURVE('',#5277,#5276,#2666,.T.);
#6541=EDGE_CURVE('',#5278,#5277,#4401,.T.);
#6542=EDGE_CURVE('',#5279,#5278,#2667,.T.);
#6543=EDGE_CURVE('',#5280,#5279,#4402,.T.);
#6544=EDGE_CURVE('',#5281,#5280,#2668,.T.);
#6545=EDGE_CURVE('',#5282,#5281,#2669,.T.);
#6546=EDGE_CURVE('',#5283,#5282,#2670,.T.);
#6547=EDGE_CURVE('',#5284,#5283,#2671,.T.);
#6548=EDGE_CURVE('',#5285,#5284,#2672,.T.);
#6549=EDGE_CURVE('',#5286,#5285,#2673,.T.);
#6550=EDGE_CURVE('',#5287,#5286,#2674,.T.);
#6551=EDGE_CURVE('',#5288,#5287,#2675,.T.);
#6552=EDGE_CURVE('',#5289,#5288,#4403,.T.);
#6553=EDGE_CURVE('',#5290,#5289,#2676,.T.);
#6554=EDGE_CURVE('',#5291,#5290,#4404,.T.);
#6555=EDGE_CURVE('',#5292,#5291,#2677,.T.);
#6556=EDGE_CURVE('',#5293,#5292,#4405,.T.);
#6557=EDGE_CURVE('',#5294,#5293,#2678,.T.);
#6558=EDGE_CURVE('',#5295,#5294,#4406,.T.);
#6559=EDGE_CURVE('',#5296,#5295,#2679,.T.);
#6560=EDGE_CURVE('',#5297,#5296,#4407,.T.);
#6561=EDGE_CURVE('',#5298,#5297,#2680,.T.);
#6562=EDGE_CURVE('',#5299,#5298,#4408,.T.);
#6563=EDGE_CURVE('',#5300,#5299,#2681,.T.);
#6564=EDGE_CURVE('',#5301,#5300,#4409,.T.);
#6565=EDGE_CURVE('',#5302,#5301,#2682,.T.);
#6566=EDGE_CURVE('',#5303,#5302,#4410,.T.);
#6567=EDGE_CURVE('',#5304,#5303,#2683,.T.);
#6568=EDGE_CURVE('',#5305,#5304,#4411,.T.);
#6569=EDGE_CURVE('',#5306,#5305,#2684,.T.);
#6570=EDGE_CURVE('',#5307,#5306,#4412,.T.);
#6571=EDGE_CURVE('',#5308,#5307,#2685,.T.);
#6572=EDGE_CURVE('',#5309,#5308,#4413,.T.);
#6573=EDGE_CURVE('',#5310,#5309,#2686,.T.);
#6574=EDGE_CURVE('',#5311,#5310,#2687,.T.);
#6575=EDGE_CURVE('',#5312,#5311,#2688,.T.);
#6576=EDGE_CURVE('',#5313,#5312,#2689,.T.);
#6577=EDGE_CURVE('',#5314,#5313,#2690,.T.);
#6578=EDGE_CURVE('',#5315,#5314,#2691,.T.);
#6579=EDGE_CURVE('',#5316,#5315,#2692,.T.);
#6580=EDGE_CURVE('',#5317,#5316,#2693,.T.);
#6581=EDGE_CURVE('',#5318,#5317,#4414,.T.);
#6582=EDGE_CURVE('',#5319,#5318,#2694,.T.);
#6583=EDGE_CURVE('',#5320,#5319,#4415,.T.);
#6584=EDGE_CURVE('',#5321,#5320,#2695,.T.);
#6585=EDGE_CURVE('',#5322,#5321,#4416,.T.);
#6586=EDGE_CURVE('',#5323,#5322,#2696,.T.);
#6587=EDGE_CURVE('',#5324,#5323,#4417,.T.);
#6588=EDGE_CURVE('',#5325,#5324,#2697,.T.);
#6589=EDGE_CURVE('',#5326,#5325,#4418,.T.);
#6590=EDGE_CURVE('',#5327,#5326,#2698,.T.);
#6591=EDGE_CURVE('',#5328,#5327,#4419,.T.);
#6592=EDGE_CURVE('',#5329,#5328,#2699,.T.);
#6593=EDGE_CURVE('',#5330,#5329,#4420,.T.);
#6594=EDGE_CURVE('',#5331,#5330,#2700,.T.);
#6595=EDGE_CURVE('',#5332,#5331,#4421,.T.);
#6596=EDGE_CURVE('',#5333,#5332,#2701,.T.);
#6597=EDGE_CURVE('',#5334,#5333,#4422,.T.);
#6598=EDGE_CURVE('',#5335,#5334,#2702,.T.);
#6599=EDGE_CURVE('',#5336,#5335,#4423,.T.);
#6600=EDGE_CURVE('',#5337,#5336,#2703,.T.);
#6601=EDGE_CURVE('',#5338,#5337,#4424,.T.);
#6602=EDGE_CURVE('',#5339,#5338,#2704,.T.);
#6603=EDGE_CURVE('',#5340,#5339,#2705,.T.);
#6604=EDGE_CURVE('',#5341,#5340,#2706,.T.);
#6605=EDGE_CURVE('',#5227,#5341,#2707,.T.);
#6606=EDGE_CURVE('',#5342,#5343,#4425,.T.);
#6607=EDGE_CURVE('',#5343,#5344,#2708,.T.);
#6608=EDGE_CURVE('',#5344,#5345,#4426,.T.);
#6609=EDGE_CURVE('',#5345,#5346,#2709,.T.);
#6610=EDGE_CURVE('',#5346,#5347,#4427,.T.);
#6611=EDGE_CURVE('',#5347,#5348,#2710,.T.);
#6612=EDGE_CURVE('',#5348,#5349,#4428,.T.);
#6613=EDGE_CURVE('',#5349,#5342,#2711,.T.);
#6614=EDGE_CURVE('',#5350,#5351,#4429,.T.);
#6615=EDGE_CURVE('',#5351,#5352,#2712,.T.);
#6616=EDGE_CURVE('',#5352,#5353,#4430,.T.);
#6617=EDGE_CURVE('',#5353,#5354,#2713,.T.);
#6618=EDGE_CURVE('',#5354,#5355,#4431,.T.);
#6619=EDGE_CURVE('',#5355,#5356,#2714,.T.);
#6620=EDGE_CURVE('',#5356,#5357,#4432,.T.);
#6621=EDGE_CURVE('',#5357,#5350,#2715,.T.);
#6622=EDGE_CURVE('',#5358,#5359,#4433,.T.);
#6623=EDGE_CURVE('',#5359,#5360,#2716,.T.);
#6624=EDGE_CURVE('',#5360,#5361,#4434,.T.);
#6625=EDGE_CURVE('',#5361,#5362,#2717,.T.);
#6626=EDGE_CURVE('',#5362,#5363,#4435,.T.);
#6627=EDGE_CURVE('',#5363,#5364,#2718,.T.);
#6628=EDGE_CURVE('',#5364,#5365,#4436,.T.);
#6629=EDGE_CURVE('',#5365,#5358,#2719,.T.);
#6630=EDGE_CURVE('',#5366,#5367,#4437,.T.);
#6631=EDGE_CURVE('',#5367,#5368,#2720,.T.);
#6632=EDGE_CURVE('',#5368,#5369,#4438,.T.);
#6633=EDGE_CURVE('',#5369,#5370,#2721,.T.);
#6634=EDGE_CURVE('',#5370,#5371,#4439,.T.);
#6635=EDGE_CURVE('',#5371,#5372,#2722,.T.);
#6636=EDGE_CURVE('',#5372,#5373,#4440,.T.);
#6637=EDGE_CURVE('',#5373,#5366,#2723,.T.);
#6638=EDGE_CURVE('',#5374,#5375,#4441,.T.);
#6639=EDGE_CURVE('',#5375,#5376,#2724,.T.);
#6640=EDGE_CURVE('',#5376,#5377,#4442,.T.);
#6641=EDGE_CURVE('',#5377,#5063,#2725,.T.);
#6642=EDGE_CURVE('',#5062,#5378,#2726,.T.);
#6643=EDGE_CURVE('',#5378,#5379,#4443,.T.);
#6644=EDGE_CURVE('',#5379,#5380,#2727,.T.);
#6645=EDGE_CURVE('',#5380,#5381,#4444,.T.);
#6646=EDGE_CURVE('',#5381,#5382,#2728,.T.);
#6647=EDGE_CURVE('',#5382,#5383,#4445,.T.);
#6648=EDGE_CURVE('',#5383,#5384,#2729,.T.);
#6649=EDGE_CURVE('',#5384,#5385,#4446,.T.);
#6650=EDGE_CURVE('',#5385,#5386,#2730,.T.);
#6651=EDGE_CURVE('',#5386,#5387,#4447,.T.);
#6652=EDGE_CURVE('',#5387,#5374,#2731,.T.);
#6653=EDGE_CURVE('',#5065,#5227,#2732,.T.);
#6654=EDGE_CURVE('',#5064,#5226,#2733,.T.);
#6655=EDGE_CURVE('',#5066,#5341,#2734,.T.);
#6656=EDGE_CURVE('',#5067,#5340,#2735,.T.);
#6657=EDGE_CURVE('',#5068,#5339,#2736,.T.);
#6658=EDGE_CURVE('',#5069,#5338,#2737,.T.);
#6659=EDGE_CURVE('',#5070,#5337,#2738,.T.);
#6660=EDGE_CURVE('',#5071,#5336,#2739,.T.);
#6661=EDGE_CURVE('',#5072,#5335,#2740,.T.);
#6662=EDGE_CURVE('',#5073,#5334,#2741,.T.);
#6663=EDGE_CURVE('',#5074,#5333,#2742,.T.);
#6664=EDGE_CURVE('',#5075,#5332,#2743,.T.);
#6665=EDGE_CURVE('',#5076,#5331,#2744,.T.);
#6666=EDGE_CURVE('',#5077,#5330,#2745,.T.);
#6667=EDGE_CURVE('',#5078,#5329,#2746,.T.);
#6668=EDGE_CURVE('',#5079,#5328,#2747,.T.);
#6669=EDGE_CURVE('',#5080,#5327,#2748,.T.);
#6670=EDGE_CURVE('',#5081,#5326,#2749,.T.);
#6671=EDGE_CURVE('',#5082,#5325,#2750,.T.);
#6672=EDGE_CURVE('',#5083,#5324,#2751,.T.);
#6673=EDGE_CURVE('',#5084,#5323,#2752,.T.);
#6674=EDGE_CURVE('',#5085,#5322,#2753,.T.);
#6675=EDGE_CURVE('',#5086,#5321,#2754,.T.);
#6676=EDGE_CURVE('',#5087,#5320,#2755,.T.);
#6677=EDGE_CURVE('',#5088,#5319,#2756,.T.);
#6678=EDGE_CURVE('',#5089,#5318,#2757,.T.);
#6679=EDGE_CURVE('',#5090,#5317,#2758,.T.);
#6680=EDGE_CURVE('',#5091,#5316,#2759,.T.);
#6681=EDGE_CURVE('',#5092,#5315,#2760,.T.);
#6682=EDGE_CURVE('',#5093,#5314,#2761,.T.);
#6683=EDGE_CURVE('',#5094,#5313,#2762,.T.);
#6684=EDGE_CURVE('',#5095,#5312,#2763,.T.);
#6685=EDGE_CURVE('',#5096,#5311,#2764,.T.);
#6686=EDGE_CURVE('',#5097,#5310,#2765,.T.);
#6687=EDGE_CURVE('',#5098,#5309,#2766,.T.);
#6688=EDGE_CURVE('',#5099,#5308,#2767,.T.);
#6689=EDGE_CURVE('',#5100,#5307,#2768,.T.);
#6690=EDGE_CURVE('',#5101,#5306,#2769,.T.);
#6691=EDGE_CURVE('',#5102,#5305,#2770,.T.);
#6692=EDGE_CURVE('',#5103,#5304,#2771,.T.);
#6693=EDGE_CURVE('',#5104,#5303,#2772,.T.);
#6694=EDGE_CURVE('',#5105,#5302,#2773,.T.);
#6695=EDGE_CURVE('',#5106,#5301,#2774,.T.);
#6696=EDGE_CURVE('',#5107,#5300,#2775,.T.);
#6697=EDGE_CURVE('',#5108,#5299,#2776,.T.);
#6698=EDGE_CURVE('',#5109,#5298,#2777,.T.);
#6699=EDGE_CURVE('',#5110,#5297,#2778,.T.);
#6700=EDGE_CURVE('',#5111,#5296,#2779,.T.);
#6701=EDGE_CURVE('',#5112,#5295,#2780,.T.);
#6702=EDGE_CURVE('',#5113,#5294,#2781,.T.);
#6703=EDGE_CURVE('',#5114,#5293,#2782,.T.);
#6704=EDGE_CURVE('',#5115,#5292,#2783,.T.);
#6705=EDGE_CURVE('',#5116,#5291,#2784,.T.);
#6706=EDGE_CURVE('',#5117,#5290,#2785,.T.);
#6707=EDGE_CURVE('',#5118,#5289,#2786,.T.);
#6708=EDGE_CURVE('',#5119,#5288,#2787,.T.);
#6709=EDGE_CURVE('',#5120,#5287,#2788,.T.);
#6710=EDGE_CURVE('',#5121,#5286,#2789,.T.);
#6711=EDGE_CURVE('',#5122,#5285,#2790,.T.);
#6712=EDGE_CURVE('',#5123,#5284,#2791,.T.);
#6713=EDGE_CURVE('',#5124,#5283,#2792,.T.);
#6714=EDGE_CURVE('',#5125,#5282,#2793,.T.);
#6715=EDGE_CURVE('',#5126,#5281,#2794,.T.);
#6716=EDGE_CURVE('',#5127,#5280,#2795,.T.);
#6717=EDGE_CURVE('',#5128,#5279,#2796,.T.);
#6718=EDGE_CURVE('',#5129,#5278,#2797,.T.);
#6719=EDGE_CURVE('',#5130,#5277,#2798,.T.);
#6720=EDGE_CURVE('',#5131,#5276,#2799,.T.);
#6721=EDGE_CURVE('',#5132,#5275,#2800,.T.);
#6722=EDGE_CURVE('',#5133,#5274,#2801,.T.);
#6723=EDGE_CURVE('',#5134,#5273,#2802,.T.);
#6724=EDGE_CURVE('',#5135,#5272,#2803,.T.);
#6725=EDGE_CURVE('',#5136,#5271,#2804,.T.);
#6726=EDGE_CURVE('',#5137,#5270,#2805,.T.);
#6727=EDGE_CURVE('',#5138,#5269,#2806,.T.);
#6728=EDGE_CURVE('',#5139,#5268,#2807,.T.);
#6729=EDGE_CURVE('',#5140,#5267,#2808,.T.);
#6730=EDGE_CURVE('',#5141,#5266,#2809,.T.);
#6731=EDGE_CURVE('',#5142,#5265,#2810,.T.);
#6732=EDGE_CURVE('',#5143,#5264,#2811,.T.);
#6733=EDGE_CURVE('',#5144,#5263,#2812,.T.);
#6734=EDGE_CURVE('',#5145,#5262,#2813,.T.);
#6735=EDGE_CURVE('',#5146,#5261,#2814,.T.);
#6736=EDGE_CURVE('',#5147,#5260,#2815,.T.);
#6737=EDGE_CURVE('',#5148,#5259,#2816,.T.);
#6738=EDGE_CURVE('',#5149,#5258,#2817,.T.);
#6739=EDGE_CURVE('',#5150,#5257,#2818,.T.);
#6740=EDGE_CURVE('',#5151,#5256,#2819,.T.);
#6741=EDGE_CURVE('',#5152,#5255,#2820,.T.);
#6742=EDGE_CURVE('',#5153,#5254,#2821,.T.);
#6743=EDGE_CURVE('',#5154,#5253,#2822,.T.);
#6744=EDGE_CURVE('',#5155,#5252,#2823,.T.);
#6745=EDGE_CURVE('',#5156,#5251,#2824,.T.);
#6746=EDGE_CURVE('',#5157,#5250,#2825,.T.);
#6747=EDGE_CURVE('',#5158,#5249,#2826,.T.);
#6748=EDGE_CURVE('',#5159,#5248,#2827,.T.);
#6749=EDGE_CURVE('',#5160,#5247,#2828,.T.);
#6750=EDGE_CURVE('',#5161,#5246,#2829,.T.);
#6751=EDGE_CURVE('',#5162,#5245,#2830,.T.);
#6752=EDGE_CURVE('',#5163,#5244,#2831,.T.);
#6753=EDGE_CURVE('',#5164,#5243,#2832,.T.);
#6754=EDGE_CURVE('',#5165,#5242,#2833,.T.);
#6755=EDGE_CURVE('',#5166,#5241,#2834,.T.);
#6756=EDGE_CURVE('',#5167,#5240,#2835,.T.);
#6757=EDGE_CURVE('',#5168,#5239,#2836,.T.);
#6758=EDGE_CURVE('',#5169,#5238,#2837,.T.);
#6759=EDGE_CURVE('',#5170,#5237,#2838,.T.);
#6760=EDGE_CURVE('',#5171,#5236,#2839,.T.);
#6761=EDGE_CURVE('',#5172,#5235,#2840,.T.);
#6762=EDGE_CURVE('',#5173,#5234,#2841,.T.);
#6763=EDGE_CURVE('',#5174,#5233,#2842,.T.);
#6764=EDGE_CURVE('',#5175,#5232,#2843,.T.);
#6765=EDGE_CURVE('',#5176,#5231,#2844,.T.);
#6766=EDGE_CURVE('',#5177,#5230,#2845,.T.);
#6767=EDGE_CURVE('',#5178,#5229,#2846,.T.);
#6768=EDGE_CURVE('',#5179,#5228,#2847,.T.);
#6769=EDGE_CURVE('',#5182,#5342,#2848,.T.);
#6770=EDGE_CURVE('',#5180,#5343,#2849,.T.);
#6771=EDGE_CURVE('',#5181,#5344,#2850,.T.);
#6772=EDGE_CURVE('',#5187,#5345,#2851,.T.);
#6773=EDGE_CURVE('',#5186,#5346,#2852,.T.);
#6774=EDGE_CURVE('',#5185,#5347,#2853,.T.);
#6775=EDGE_CURVE('',#5184,#5348,#2854,.T.);
#6776=EDGE_CURVE('',#5183,#5349,#2855,.T.);
#6777=EDGE_CURVE('',#5190,#5374,#2856,.T.);
#6778=EDGE_CURVE('',#5188,#5375,#2857,.T.);
#6779=EDGE_CURVE('',#5189,#5376,#2858,.T.);
#6780=EDGE_CURVE('',#5201,#5377,#2859,.T.);
#6781=EDGE_CURVE('',#5200,#5378,#2860,.T.);
#6782=EDGE_CURVE('',#5199,#5379,#2861,.T.);
#6783=EDGE_CURVE('',#5198,#5380,#2862,.T.);
#6784=EDGE_CURVE('',#5197,#5381,#2863,.T.);
#6785=EDGE_CURVE('',#5196,#5382,#2864,.T.);
#6786=EDGE_CURVE('',#5195,#5383,#2865,.T.);
#6787=EDGE_CURVE('',#5194,#5384,#2866,.T.);
#6788=EDGE_CURVE('',#5193,#5385,#2867,.T.);
#6789=EDGE_CURVE('',#5192,#5386,#2868,.T.);
#6790=EDGE_CURVE('',#5191,#5387,#2869,.T.);
#6791=EDGE_CURVE('',#5204,#5350,#2870,.T.);
#6792=EDGE_CURVE('',#5202,#5351,#2871,.T.);
#6793=EDGE_CURVE('',#5203,#5352,#2872,.T.);
#6794=EDGE_CURVE('',#5209,#5353,#2873,.T.);
#6795=EDGE_CURVE('',#5208,#5354,#2874,.T.);
#6796=EDGE_CURVE('',#5207,#5355,#2875,.T.);
#6797=EDGE_CURVE('',#5206,#5356,#2876,.T.);
#6798=EDGE_CURVE('',#5205,#5357,#2877,.T.);
#6799=EDGE_CURVE('',#5212,#5366,#2878,.T.);
#6800=EDGE_CURVE('',#5210,#5367,#2879,.T.);
#6801=EDGE_CURVE('',#5211,#5368,#2880,.T.);
#6802=EDGE_CURVE('',#5217,#5369,#2881,.T.);
#6803=EDGE_CURVE('',#5216,#5370,#2882,.T.);
#6804=EDGE_CURVE('',#5215,#5371,#2883,.T.);
#6805=EDGE_CURVE('',#5214,#5372,#2884,.T.);
#6806=EDGE_CURVE('',#5213,#5373,#2885,.T.);
#6807=EDGE_CURVE('',#5220,#5358,#2886,.T.);
#6808=EDGE_CURVE('',#5218,#5359,#2887,.T.);
#6809=EDGE_CURVE('',#5219,#5360,#2888,.T.);
#6810=EDGE_CURVE('',#5225,#5361,#2889,.T.);
#6811=EDGE_CURVE('',#5224,#5362,#2890,.T.);
#6812=EDGE_CURVE('',#5223,#5363,#2891,.T.);
#6813=EDGE_CURVE('',#5222,#5364,#2892,.T.);
#6814=EDGE_CURVE('',#5221,#5365,#2893,.T.);
#8580=ORIENTED_EDGE('',*,*,#6323,.T.);
#8581=ORIENTED_EDGE('',*,*,#6324,.T.);
#8582=ORIENTED_EDGE('',*,*,#6325,.F.);
#8583=ORIENTED_EDGE('',*,*,#6326,.F.);
#8584=ORIENTED_EDGE('',*,*,#6327,.T.);
#8585=ORIENTED_EDGE('',*,*,#6328,.T.);
#8586=ORIENTED_EDGE('',*,*,#6329,.T.);
#8587=ORIENTED_EDGE('',*,*,#6330,.T.);
#8588=ORIENTED_EDGE('',*,*,#6331,.T.);
#8589=ORIENTED_EDGE('',*,*,#6332,.T.);
#8590=ORIENTED_EDGE('',*,*,#6333,.T.);
#8591=ORIENTED_EDGE('',*,*,#6334,.T.);
#8592=ORIENTED_EDGE('',*,*,#6335,.T.);
#8593=ORIENTED_EDGE('',*,*,#6336,.T.);
#8594=ORIENTED_EDGE('',*,*,#6337,.T.);
#8595=ORIENTED_EDGE('',*,*,#6338,.T.);
#8596=ORIENTED_EDGE('',*,*,#6339,.T.);
#8597=ORIENTED_EDGE('',*,*,#6340,.T.);
#8598=ORIENTED_EDGE('',*,*,#6341,.T.);
#8599=ORIENTED_EDGE('',*,*,#6342,.T.);
#8600=ORIENTED_EDGE('',*,*,#6343,.T.);
#8601=ORIENTED_EDGE('',*,*,#6344,.T.);
#8602=ORIENTED_EDGE('',*,*,#6345,.T.);
#8603=ORIENTED_EDGE('',*,*,#6346,.T.);
#8604=ORIENTED_EDGE('',*,*,#6347,.T.);
#8605=ORIENTED_EDGE('',*,*,#6348,.T.);
#8606=ORIENTED_EDGE('',*,*,#6349,.T.);
#8607=ORIENTED_EDGE('',*,*,#6350,.T.);
#8608=ORIENTED_EDGE('',*,*,#6351,.T.);
#8609=ORIENTED_EDGE('',*,*,#6352,.T.);
#8610=ORIENTED_EDGE('',*,*,#6353,.T.);
#8611=ORIENTED_EDGE('',*,*,#6354,.T.);
#8612=ORIENTED_EDGE('',*,*,#6355,.T.);
#8613=ORIENTED_EDGE('',*,*,#6356,.T.);
#8614=ORIENTED_EDGE('',*,*,#6357,.T.);
#8615=ORIENTED_EDGE('',*,*,#6358,.T.);
#8616=ORIENTED_EDGE('',*,*,#6359,.T.);
#8617=ORIENTED_EDGE('',*,*,#6360,.T.);
#8618=ORIENTED_EDGE('',*,*,#6361,.T.);
#8619=ORIENTED_EDGE('',*,*,#6362,.T.);
#8620=ORIENTED_EDGE('',*,*,#6363,.T.);
#8621=ORIENTED_EDGE('',*,*,#6364,.T.);
#8622=ORIENTED_EDGE('',*,*,#6365,.T.);
#8623=ORIENTED_EDGE('',*,*,#6366,.T.);
#8624=ORIENTED_EDGE('',*,*,#6367,.T.);
#8625=ORIENTED_EDGE('',*,*,#6368,.T.);
#8626=ORIENTED_EDGE('',*,*,#6369,.T.);
#8627=ORIENTED_EDGE('',*,*,#6370,.T.);
#8628=ORIENTED_EDGE('',*,*,#6371,.T.);
#8629=ORIENTED_EDGE('',*,*,#6372,.T.);
#8630=ORIENTED_EDGE('',*,*,#6373,.T.);
#8631=ORIENTED_EDGE('',*,*,#6374,.T.);
#8632=ORIENTED_EDGE('',*,*,#6375,.T.);
#8633=ORIENTED_EDGE('',*,*,#6376,.T.);
#8634=ORIENTED_EDGE('',*,*,#6377,.T.);
#8635=ORIENTED_EDGE('',*,*,#6378,.T.);
#8636=ORIENTED_EDGE('',*,*,#6379,.T.);
#8637=ORIENTED_EDGE('',*,*,#6380,.T.);
#8638=ORIENTED_EDGE('',*,*,#6381,.T.);
#8639=ORIENTED_EDGE('',*,*,#6382,.T.);
#8640=ORIENTED_EDGE('',*,*,#6383,.T.);
#8641=ORIENTED_EDGE('',*,*,#6384,.T.);
#8642=ORIENTED_EDGE('',*,*,#6385,.T.);
#8643=ORIENTED_EDGE('',*,*,#6386,.T.);
#8644=ORIENTED_EDGE('',*,*,#6387,.T.);
#8645=ORIENTED_EDGE('',*,*,#6388,.T.);
#8646=ORIENTED_EDGE('',*,*,#6389,.T.);
#8647=ORIENTED_EDGE('',*,*,#6390,.T.);
#8648=ORIENTED_EDGE('',*,*,#6391,.T.);
#8649=ORIENTED_EDGE('',*,*,#6392,.T.);
#8650=ORIENTED_EDGE('',*,*,#6393,.T.);
#8651=ORIENTED_EDGE('',*,*,#6394,.T.);
#8652=ORIENTED_EDGE('',*,*,#6395,.T.);
#8653=ORIENTED_EDGE('',*,*,#6396,.T.);
#8654=ORIENTED_EDGE('',*,*,#6397,.T.);
#8655=ORIENTED_EDGE('',*,*,#6398,.T.);
#8656=ORIENTED_EDGE('',*,*,#6399,.T.);
#8657=ORIENTED_EDGE('',*,*,#6400,.T.);
#8658=ORIENTED_EDGE('',*,*,#6401,.T.);
#8659=ORIENTED_EDGE('',*,*,#6402,.T.);
#8660=ORIENTED_EDGE('',*,*,#6403,.T.);
#8661=ORIENTED_EDGE('',*,*,#6404,.T.);
#8662=ORIENTED_EDGE('',*,*,#6405,.T.);
#8663=ORIENTED_EDGE('',*,*,#6406,.T.);
#8664=ORIENTED_EDGE('',*,*,#6407,.T.);
#8665=ORIENTED_EDGE('',*,*,#6408,.T.);
#8666=ORIENTED_EDGE('',*,*,#6409,.T.);
#8667=ORIENTED_EDGE('',*,*,#6410,.T.);
#8668=ORIENTED_EDGE('',*,*,#6411,.T.);
#8669=ORIENTED_EDGE('',*,*,#6412,.T.);
#8670=ORIENTED_EDGE('',*,*,#6413,.T.);
#8671=ORIENTED_EDGE('',*,*,#6414,.T.);
#8672=ORIENTED_EDGE('',*,*,#6415,.T.);
#8673=ORIENTED_EDGE('',*,*,#6416,.T.);
#8674=ORIENTED_EDGE('',*,*,#6417,.T.);
#8675=ORIENTED_EDGE('',*,*,#6418,.T.);
#8676=ORIENTED_EDGE('',*,*,#6419,.T.);
#8677=ORIENTED_EDGE('',*,*,#6420,.T.);
#8678=ORIENTED_EDGE('',*,*,#6421,.T.);
#8679=ORIENTED_EDGE('',*,*,#6422,.T.);
#8680=ORIENTED_EDGE('',*,*,#6423,.T.);
#8681=ORIENTED_EDGE('',*,*,#6424,.T.);
#8682=ORIENTED_EDGE('',*,*,#6425,.T.);
#8683=ORIENTED_EDGE('',*,*,#6426,.T.);
#8684=ORIENTED_EDGE('',*,*,#6427,.T.);
#8685=ORIENTED_EDGE('',*,*,#6428,.T.);
#8686=ORIENTED_EDGE('',*,*,#6429,.T.);
#8687=ORIENTED_EDGE('',*,*,#6430,.T.);
#8688=ORIENTED_EDGE('',*,*,#6431,.T.);
#8689=ORIENTED_EDGE('',*,*,#6432,.T.);
#8690=ORIENTED_EDGE('',*,*,#6433,.T.);
#8691=ORIENTED_EDGE('',*,*,#6434,.T.);
#8692=ORIENTED_EDGE('',*,*,#6435,.T.);
#8693=ORIENTED_EDGE('',*,*,#6436,.T.);
#8694=ORIENTED_EDGE('',*,*,#6437,.T.);
#8695=ORIENTED_EDGE('',*,*,#6438,.T.);
#8696=ORIENTED_EDGE('',*,*,#6439,.T.);
#8697=ORIENTED_EDGE('',*,*,#6440,.T.);
#8698=ORIENTED_EDGE('',*,*,#6441,.T.);
#8699=ORIENTED_EDGE('',*,*,#6442,.T.);
#8700=ORIENTED_EDGE('',*,*,#6443,.F.);
#8701=ORIENTED_EDGE('',*,*,#6444,.F.);
#8702=ORIENTED_EDGE('',*,*,#6445,.F.);
#8703=ORIENTED_EDGE('',*,*,#6446,.F.);
#8704=ORIENTED_EDGE('',*,*,#6447,.F.);
#8705=ORIENTED_EDGE('',*,*,#6448,.F.);
#8706=ORIENTED_EDGE('',*,*,#6449,.F.);
#8707=ORIENTED_EDGE('',*,*,#6450,.F.);
#8708=ORIENTED_EDGE('',*,*,#6451,.F.);
#8709=ORIENTED_EDGE('',*,*,#6452,.F.);
#8710=ORIENTED_EDGE('',*,*,#6453,.F.);
#8711=ORIENTED_EDGE('',*,*,#6454,.F.);
#8712=ORIENTED_EDGE('',*,*,#6455,.F.);
#8713=ORIENTED_EDGE('',*,*,#6456,.F.);
#8714=ORIENTED_EDGE('',*,*,#6457,.F.);
#8715=ORIENTED_EDGE('',*,*,#6458,.F.);
#8716=ORIENTED_EDGE('',*,*,#6459,.F.);
#8717=ORIENTED_EDGE('',*,*,#6460,.F.);
#8718=ORIENTED_EDGE('',*,*,#6461,.F.);
#8719=ORIENTED_EDGE('',*,*,#6462,.F.);
#8720=ORIENTED_EDGE('',*,*,#6463,.F.);
#8721=ORIENTED_EDGE('',*,*,#6323,.F.);
#8722=ORIENTED_EDGE('',*,*,#6464,.F.);
#8723=ORIENTED_EDGE('',*,*,#6465,.F.);
#8724=ORIENTED_EDGE('',*,*,#6466,.F.);
#8725=ORIENTED_EDGE('',*,*,#6467,.F.);
#8726=ORIENTED_EDGE('',*,*,#6468,.F.);
#8727=ORIENTED_EDGE('',*,*,#6469,.F.);
#8728=ORIENTED_EDGE('',*,*,#6470,.F.);
#8729=ORIENTED_EDGE('',*,*,#6471,.F.);
#8730=ORIENTED_EDGE('',*,*,#6472,.F.);
#8731=ORIENTED_EDGE('',*,*,#6473,.F.);
#8732=ORIENTED_EDGE('',*,*,#6474,.F.);
#8733=ORIENTED_EDGE('',*,*,#6475,.F.);
#8734=ORIENTED_EDGE('',*,*,#6476,.F.);
#8735=ORIENTED_EDGE('',*,*,#6477,.F.);
#8736=ORIENTED_EDGE('',*,*,#6478,.F.);
#8737=ORIENTED_EDGE('',*,*,#6479,.F.);
#8738=ORIENTED_EDGE('',*,*,#6480,.F.);
#8739=ORIENTED_EDGE('',*,*,#6481,.F.);
#8740=ORIENTED_EDGE('',*,*,#6482,.F.);
#8741=ORIENTED_EDGE('',*,*,#6483,.F.);
#8742=ORIENTED_EDGE('',*,*,#6484,.F.);
#8743=ORIENTED_EDGE('',*,*,#6485,.F.);
#8744=ORIENTED_EDGE('',*,*,#6486,.F.);
#8745=ORIENTED_EDGE('',*,*,#6487,.F.);
#8746=ORIENTED_EDGE('',*,*,#6488,.F.);
#8747=ORIENTED_EDGE('',*,*,#6489,.F.);
#8748=ORIENTED_EDGE('',*,*,#6490,.F.);
#8749=ORIENTED_EDGE('',*,*,#6491,.F.);
#8750=ORIENTED_EDGE('',*,*,#6492,.F.);
#8751=ORIENTED_EDGE('',*,*,#6493,.F.);
#8752=ORIENTED_EDGE('',*,*,#6494,.F.);
#8753=ORIENTED_EDGE('',*,*,#6495,.F.);
#8754=ORIENTED_EDGE('',*,*,#6496,.F.);
#8755=ORIENTED_EDGE('',*,*,#6497,.F.);
#8756=ORIENTED_EDGE('',*,*,#6498,.F.);
#8757=ORIENTED_EDGE('',*,*,#6499,.F.);
#8758=ORIENTED_EDGE('',*,*,#6500,.F.);
#8759=ORIENTED_EDGE('',*,*,#6501,.F.);
#8760=ORIENTED_EDGE('',*,*,#6502,.F.);
#8761=ORIENTED_EDGE('',*,*,#6503,.F.);
#8762=ORIENTED_EDGE('',*,*,#6504,.F.);
#8763=ORIENTED_EDGE('',*,*,#6505,.F.);
#8764=ORIENTED_EDGE('',*,*,#6506,.F.);
#8765=ORIENTED_EDGE('',*,*,#6507,.F.);
#8766=ORIENTED_EDGE('',*,*,#6508,.F.);
#8767=ORIENTED_EDGE('',*,*,#6509,.F.);
#8768=ORIENTED_EDGE('',*,*,#6510,.F.);
#8769=ORIENTED_EDGE('',*,*,#6511,.F.);
#8770=ORIENTED_EDGE('',*,*,#6512,.F.);
#8771=ORIENTED_EDGE('',*,*,#6513,.F.);
#8772=ORIENTED_EDGE('',*,*,#6514,.F.);
#8773=ORIENTED_EDGE('',*,*,#6515,.F.);
#8774=ORIENTED_EDGE('',*,*,#6516,.F.);
#8775=ORIENTED_EDGE('',*,*,#6517,.F.);
#8776=ORIENTED_EDGE('',*,*,#6518,.F.);
#8777=ORIENTED_EDGE('',*,*,#6519,.F.);
#8778=ORIENTED_EDGE('',*,*,#6520,.F.);
#8779=ORIENTED_EDGE('',*,*,#6521,.F.);
#8780=ORIENTED_EDGE('',*,*,#6522,.F.);
#8781=ORIENTED_EDGE('',*,*,#6523,.F.);
#8782=ORIENTED_EDGE('',*,*,#6524,.F.);
#8783=ORIENTED_EDGE('',*,*,#6525,.F.);
#8784=ORIENTED_EDGE('',*,*,#6526,.F.);
#8785=ORIENTED_EDGE('',*,*,#6527,.F.);
#8786=ORIENTED_EDGE('',*,*,#6528,.F.);
#8787=ORIENTED_EDGE('',*,*,#6529,.F.);
#8788=ORIENTED_EDGE('',*,*,#6530,.F.);
#8789=ORIENTED_EDGE('',*,*,#6531,.F.);
#8790=ORIENTED_EDGE('',*,*,#6532,.F.);
#8791=ORIENTED_EDGE('',*,*,#6533,.F.);
#8792=ORIENTED_EDGE('',*,*,#6534,.F.);
#8793=ORIENTED_EDGE('',*,*,#6535,.F.);
#8794=ORIENTED_EDGE('',*,*,#6536,.F.);
#8795=ORIENTED_EDGE('',*,*,#6537,.F.);
#8796=ORIENTED_EDGE('',*,*,#6538,.F.);
#8797=ORIENTED_EDGE('',*,*,#6539,.F.);
#8798=ORIENTED_EDGE('',*,*,#6540,.F.);
#8799=ORIENTED_EDGE('',*,*,#6541,.F.);
#8800=ORIENTED_EDGE('',*,*,#6542,.F.);
#8801=ORIENTED_EDGE('',*,*,#6543,.F.);
#8802=ORIENTED_EDGE('',*,*,#6544,.F.);
#8803=ORIENTED_EDGE('',*,*,#6545,.F.);
#8804=ORIENTED_EDGE('',*,*,#6546,.F.);
#8805=ORIENTED_EDGE('',*,*,#6547,.F.);
#8806=ORIENTED_EDGE('',*,*,#6548,.F.);
#8807=ORIENTED_EDGE('',*,*,#6549,.F.);
#8808=ORIENTED_EDGE('',*,*,#6550,.F.);
#8809=ORIENTED_EDGE('',*,*,#6551,.F.);
#8810=ORIENTED_EDGE('',*,*,#6552,.F.);
#8811=ORIENTED_EDGE('',*,*,#6553,.F.);
#8812=ORIENTED_EDGE('',*,*,#6554,.F.);
#8813=ORIENTED_EDGE('',*,*,#6555,.F.);
#8814=ORIENTED_EDGE('',*,*,#6556,.F.);
#8815=ORIENTED_EDGE('',*,*,#6557,.F.);
#8816=ORIENTED_EDGE('',*,*,#6558,.F.);
#8817=ORIENTED_EDGE('',*,*,#6559,.F.);
#8818=ORIENTED_EDGE('',*,*,#6560,.F.);
#8819=ORIENTED_EDGE('',*,*,#6561,.F.);
#8820=ORIENTED_EDGE('',*,*,#6562,.F.);
#8821=ORIENTED_EDGE('',*,*,#6563,.F.);
#8822=ORIENTED_EDGE('',*,*,#6564,.F.);
#8823=ORIENTED_EDGE('',*,*,#6565,.F.);
#8824=ORIENTED_EDGE('',*,*,#6566,.F.);
#8825=ORIENTED_EDGE('',*,*,#6567,.F.);
#8826=ORIENTED_EDGE('',*,*,#6568,.F.);
#8827=ORIENTED_EDGE('',*,*,#6569,.F.);
#8828=ORIENTED_EDGE('',*,*,#6570,.F.);
#8829=ORIENTED_EDGE('',*,*,#6571,.F.);
#8830=ORIENTED_EDGE('',*,*,#6572,.F.);
#8831=ORIENTED_EDGE('',*,*,#6573,.F.);
#8832=ORIENTED_EDGE('',*,*,#6574,.F.);
#8833=ORIENTED_EDGE('',*,*,#6575,.F.);
#8834=ORIENTED_EDGE('',*,*,#6576,.F.);
#8835=ORIENTED_EDGE('',*,*,#6577,.F.);
#8836=ORIENTED_EDGE('',*,*,#6578,.F.);
#8837=ORIENTED_EDGE('',*,*,#6579,.F.);
#8838=ORIENTED_EDGE('',*,*,#6580,.F.);
#8839=ORIENTED_EDGE('',*,*,#6581,.F.);
#8840=ORIENTED_EDGE('',*,*,#6582,.F.);
#8841=ORIENTED_EDGE('',*,*,#6583,.F.);
#8842=ORIENTED_EDGE('',*,*,#6584,.F.);
#8843=ORIENTED_EDGE('',*,*,#6585,.F.);
#8844=ORIENTED_EDGE('',*,*,#6586,.F.);
#8845=ORIENTED_EDGE('',*,*,#6587,.F.);
#8846=ORIENTED_EDGE('',*,*,#6588,.F.);
#8847=ORIENTED_EDGE('',*,*,#6589,.F.);
#8848=ORIENTED_EDGE('',*,*,#6590,.F.);
#8849=ORIENTED_EDGE('',*,*,#6591,.F.);
#8850=ORIENTED_EDGE('',*,*,#6592,.F.);
#8851=ORIENTED_EDGE('',*,*,#6593,.F.);
#8852=ORIENTED_EDGE('',*,*,#6594,.F.);
#8853=ORIENTED_EDGE('',*,*,#6595,.F.);
#8854=ORIENTED_EDGE('',*,*,#6596,.F.);
#8855=ORIENTED_EDGE('',*,*,#6597,.F.);
#8856=ORIENTED_EDGE('',*,*,#6598,.F.);
#8857=ORIENTED_EDGE('',*,*,#6599,.F.);
#8858=ORIENTED_EDGE('',*,*,#6600,.F.);
#8859=ORIENTED_EDGE('',*,*,#6601,.F.);
#8860=ORIENTED_EDGE('',*,*,#6602,.F.);
#8861=ORIENTED_EDGE('',*,*,#6603,.F.);
#8862=ORIENTED_EDGE('',*,*,#6604,.F.);
#8863=ORIENTED_EDGE('',*,*,#6605,.F.);
#8864=ORIENTED_EDGE('',*,*,#6606,.T.);
#8865=ORIENTED_EDGE('',*,*,#6607,.T.);
#8866=ORIENTED_EDGE('',*,*,#6608,.T.);
#8867=ORIENTED_EDGE('',*,*,#6609,.T.);
#8868=ORIENTED_EDGE('',*,*,#6610,.T.);
#8869=ORIENTED_EDGE('',*,*,#6611,.T.);
#8870=ORIENTED_EDGE('',*,*,#6612,.T.);
#8871=ORIENTED_EDGE('',*,*,#6613,.T.);
#8872=ORIENTED_EDGE('',*,*,#6614,.T.);
#8873=ORIENTED_EDGE('',*,*,#6615,.T.);
#8874=ORIENTED_EDGE('',*,*,#6616,.T.);
#8875=ORIENTED_EDGE('',*,*,#6617,.T.);
#8876=ORIENTED_EDGE('',*,*,#6618,.T.);
#8877=ORIENTED_EDGE('',*,*,#6619,.T.);
#8878=ORIENTED_EDGE('',*,*,#6620,.T.);
#8879=ORIENTED_EDGE('',*,*,#6621,.T.);
#8880=ORIENTED_EDGE('',*,*,#6622,.T.);
#8881=ORIENTED_EDGE('',*,*,#6623,.T.);
#8882=ORIENTED_EDGE('',*,*,#6624,.T.);
#8883=ORIENTED_EDGE('',*,*,#6625,.T.);
#8884=ORIENTED_EDGE('',*,*,#6626,.T.);
#8885=ORIENTED_EDGE('',*,*,#6627,.T.);
#8886=ORIENTED_EDGE('',*,*,#6628,.T.);
#8887=ORIENTED_EDGE('',*,*,#6629,.T.);
#8888=ORIENTED_EDGE('',*,*,#6630,.T.);
#8889=ORIENTED_EDGE('',*,*,#6631,.T.);
#8890=ORIENTED_EDGE('',*,*,#6632,.T.);
#8891=ORIENTED_EDGE('',*,*,#6633,.T.);
#8892=ORIENTED_EDGE('',*,*,#6634,.T.);
#8893=ORIENTED_EDGE('',*,*,#6635,.T.);
#8894=ORIENTED_EDGE('',*,*,#6636,.T.);
#8895=ORIENTED_EDGE('',*,*,#6637,.T.);
#8896=ORIENTED_EDGE('',*,*,#6638,.T.);
#8897=ORIENTED_EDGE('',*,*,#6639,.T.);
#8898=ORIENTED_EDGE('',*,*,#6640,.T.);
#8899=ORIENTED_EDGE('',*,*,#6641,.T.);
#8900=ORIENTED_EDGE('',*,*,#6325,.T.);
#8901=ORIENTED_EDGE('',*,*,#6642,.T.);
#8902=ORIENTED_EDGE('',*,*,#6643,.T.);
#8903=ORIENTED_EDGE('',*,*,#6644,.T.);
#8904=ORIENTED_EDGE('',*,*,#6645,.T.);
#8905=ORIENTED_EDGE('',*,*,#6646,.T.);
#8906=ORIENTED_EDGE('',*,*,#6647,.T.);
#8907=ORIENTED_EDGE('',*,*,#6648,.T.);
#8908=ORIENTED_EDGE('',*,*,#6649,.T.);
#8909=ORIENTED_EDGE('',*,*,#6650,.T.);
#8910=ORIENTED_EDGE('',*,*,#6651,.T.);
#8911=ORIENTED_EDGE('',*,*,#6652,.T.);
#8912=ORIENTED_EDGE('',*,*,#6490,.T.);
#8913=ORIENTED_EDGE('',*,*,#6653,.F.);
#8914=ORIENTED_EDGE('',*,*,#6327,.F.);
#8915=ORIENTED_EDGE('',*,*,#6654,.T.);
#8916=ORIENTED_EDGE('',*,*,#6605,.T.);
#8917=ORIENTED_EDGE('',*,*,#6655,.F.);
#8918=ORIENTED_EDGE('',*,*,#6328,.F.);
#8919=ORIENTED_EDGE('',*,*,#6653,.T.);
#8920=ORIENTED_EDGE('',*,*,#6604,.T.);
#8921=ORIENTED_EDGE('',*,*,#6656,.F.);
#8922=ORIENTED_EDGE('',*,*,#6329,.F.);
#8923=ORIENTED_EDGE('',*,*,#6655,.T.);
#8924=ORIENTED_EDGE('',*,*,#6603,.T.);
#8925=ORIENTED_EDGE('',*,*,#6657,.F.);
#8926=ORIENTED_EDGE('',*,*,#6330,.F.);
#8927=ORIENTED_EDGE('',*,*,#6656,.T.);
#8928=ORIENTED_EDGE('',*,*,#6602,.T.);
#8929=ORIENTED_EDGE('',*,*,#6658,.F.);
#8930=ORIENTED_EDGE('',*,*,#6331,.F.);
#8931=ORIENTED_EDGE('',*,*,#6657,.T.);
#8932=ORIENTED_EDGE('',*,*,#6601,.T.);
#8933=ORIENTED_EDGE('',*,*,#6659,.F.);
#8934=ORIENTED_EDGE('',*,*,#6332,.F.);
#8935=ORIENTED_EDGE('',*,*,#6658,.T.);
#8936=ORIENTED_EDGE('',*,*,#6600,.T.);
#8937=ORIENTED_EDGE('',*,*,#6660,.F.);
#8938=ORIENTED_EDGE('',*,*,#6333,.F.);
#8939=ORIENTED_EDGE('',*,*,#6659,.T.);
#8940=ORIENTED_EDGE('',*,*,#6599,.T.);
#8941=ORIENTED_EDGE('',*,*,#6661,.F.);
#8942=ORIENTED_EDGE('',*,*,#6334,.F.);
#8943=ORIENTED_EDGE('',*,*,#6660,.T.);
#8944=ORIENTED_EDGE('',*,*,#6598,.T.);
#8945=ORIENTED_EDGE('',*,*,#6662,.F.);
#8946=ORIENTED_EDGE('',*,*,#6335,.F.);
#8947=ORIENTED_EDGE('',*,*,#6661,.T.);
#8948=ORIENTED_EDGE('',*,*,#6597,.T.);
#8949=ORIENTED_EDGE('',*,*,#6663,.F.);
#8950=ORIENTED_EDGE('',*,*,#6336,.F.);
#8951=ORIENTED_EDGE('',*,*,#6662,.T.);
#8952=ORIENTED_EDGE('',*,*,#6596,.T.);
#8953=ORIENTED_EDGE('',*,*,#6664,.F.);
#8954=ORIENTED_EDGE('',*,*,#6337,.F.);
#8955=ORIENTED_EDGE('',*,*,#6663,.T.);
#8956=ORIENTED_EDGE('',*,*,#6595,.T.);
#8957=ORIENTED_EDGE('',*,*,#6665,.F.);
#8958=ORIENTED_EDGE('',*,*,#6338,.F.);
#8959=ORIENTED_EDGE('',*,*,#6664,.T.);
#8960=ORIENTED_EDGE('',*,*,#6594,.T.);
#8961=ORIENTED_EDGE('',*,*,#6666,.F.);
#8962=ORIENTED_EDGE('',*,*,#6339,.F.);
#8963=ORIENTED_EDGE('',*,*,#6665,.T.);
#8964=ORIENTED_EDGE('',*,*,#6593,.T.);
#8965=ORIENTED_EDGE('',*,*,#6667,.F.);
#8966=ORIENTED_EDGE('',*,*,#6340,.F.);
#8967=ORIENTED_EDGE('',*,*,#6666,.T.);
#8968=ORIENTED_EDGE('',*,*,#6592,.T.);
#8969=ORIENTED_EDGE('',*,*,#6668,.F.);
#8970=ORIENTED_EDGE('',*,*,#6341,.F.);
#8971=ORIENTED_EDGE('',*,*,#6667,.T.);
#8972=ORIENTED_EDGE('',*,*,#6591,.T.);
#8973=ORIENTED_EDGE('',*,*,#6669,.F.);
#8974=ORIENTED_EDGE('',*,*,#6342,.F.);
#8975=ORIENTED_EDGE('',*,*,#6668,.T.);
#8976=ORIENTED_EDGE('',*,*,#6590,.T.);
#8977=ORIENTED_EDGE('',*,*,#6670,.F.);
#8978=ORIENTED_EDGE('',*,*,#6343,.F.);
#8979=ORIENTED_EDGE('',*,*,#6669,.T.);
#8980=ORIENTED_EDGE('',*,*,#6589,.T.);
#8981=ORIENTED_EDGE('',*,*,#6671,.F.);
#8982=ORIENTED_EDGE('',*,*,#6344,.F.);
#8983=ORIENTED_EDGE('',*,*,#6670,.T.);
#8984=ORIENTED_EDGE('',*,*,#6588,.T.);
#8985=ORIENTED_EDGE('',*,*,#6672,.F.);
#8986=ORIENTED_EDGE('',*,*,#6345,.F.);
#8987=ORIENTED_EDGE('',*,*,#6671,.T.);
#8988=ORIENTED_EDGE('',*,*,#6587,.T.);
#8989=ORIENTED_EDGE('',*,*,#6673,.F.);
#8990=ORIENTED_EDGE('',*,*,#6346,.F.);
#8991=ORIENTED_EDGE('',*,*,#6672,.T.);
#8992=ORIENTED_EDGE('',*,*,#6586,.T.);
#8993=ORIENTED_EDGE('',*,*,#6674,.F.);
#8994=ORIENTED_EDGE('',*,*,#6347,.F.);
#8995=ORIENTED_EDGE('',*,*,#6673,.T.);
#8996=ORIENTED_EDGE('',*,*,#6585,.T.);
#8997=ORIENTED_EDGE('',*,*,#6675,.F.);
#8998=ORIENTED_EDGE('',*,*,#6348,.F.);
#8999=ORIENTED_EDGE('',*,*,#6674,.T.);
#9000=ORIENTED_EDGE('',*,*,#6584,.T.);
#9001=ORIENTED_EDGE('',*,*,#6676,.F.);
#9002=ORIENTED_EDGE('',*,*,#6349,.F.);
#9003=ORIENTED_EDGE('',*,*,#6675,.T.);
#9004=ORIENTED_EDGE('',*,*,#6583,.T.);
#9005=ORIENTED_EDGE('',*,*,#6677,.F.);
#9006=ORIENTED_EDGE('',*,*,#6350,.F.);
#9007=ORIENTED_EDGE('',*,*,#6676,.T.);
#9008=ORIENTED_EDGE('',*,*,#6582,.T.);
#9009=ORIENTED_EDGE('',*,*,#6678,.F.);
#9010=ORIENTED_EDGE('',*,*,#6351,.F.);
#9011=ORIENTED_EDGE('',*,*,#6677,.T.);
#9012=ORIENTED_EDGE('',*,*,#6581,.T.);
#9013=ORIENTED_EDGE('',*,*,#6679,.F.);
#9014=ORIENTED_EDGE('',*,*,#6352,.F.);
#9015=ORIENTED_EDGE('',*,*,#6678,.T.);
#9016=ORIENTED_EDGE('',*,*,#6580,.T.);
#9017=ORIENTED_EDGE('',*,*,#6680,.F.);
#9018=ORIENTED_EDGE('',*,*,#6353,.F.);
#9019=ORIENTED_EDGE('',*,*,#6679,.T.);
#9020=ORIENTED_EDGE('',*,*,#6579,.T.);
#9021=ORIENTED_EDGE('',*,*,#6681,.F.);
#9022=ORIENTED_EDGE('',*,*,#6354,.F.);
#9023=ORIENTED_EDGE('',*,*,#6680,.T.);
#9024=ORIENTED_EDGE('',*,*,#6578,.T.);
#9025=ORIENTED_EDGE('',*,*,#6682,.F.);
#9026=ORIENTED_EDGE('',*,*,#6355,.F.);
#9027=ORIENTED_EDGE('',*,*,#6681,.T.);
#9028=ORIENTED_EDGE('',*,*,#6577,.T.);
#9029=ORIENTED_EDGE('',*,*,#6683,.F.);
#9030=ORIENTED_EDGE('',*,*,#6356,.F.);
#9031=ORIENTED_EDGE('',*,*,#6682,.T.);
#9032=ORIENTED_EDGE('',*,*,#6576,.T.);
#9033=ORIENTED_EDGE('',*,*,#6684,.F.);
#9034=ORIENTED_EDGE('',*,*,#6357,.F.);
#9035=ORIENTED_EDGE('',*,*,#6683,.T.);
#9036=ORIENTED_EDGE('',*,*,#6575,.T.);
#9037=ORIENTED_EDGE('',*,*,#6685,.F.);
#9038=ORIENTED_EDGE('',*,*,#6358,.F.);
#9039=ORIENTED_EDGE('',*,*,#6684,.T.);
#9040=ORIENTED_EDGE('',*,*,#6574,.T.);
#9041=ORIENTED_EDGE('',*,*,#6686,.F.);
#9042=ORIENTED_EDGE('',*,*,#6359,.F.);
#9043=ORIENTED_EDGE('',*,*,#6685,.T.);
#9044=ORIENTED_EDGE('',*,*,#6573,.T.);
#9045=ORIENTED_EDGE('',*,*,#6687,.F.);
#9046=ORIENTED_EDGE('',*,*,#6360,.F.);
#9047=ORIENTED_EDGE('',*,*,#6686,.T.);
#9048=ORIENTED_EDGE('',*,*,#6572,.T.);
#9049=ORIENTED_EDGE('',*,*,#6688,.F.);
#9050=ORIENTED_EDGE('',*,*,#6361,.F.);
#9051=ORIENTED_EDGE('',*,*,#6687,.T.);
#9052=ORIENTED_EDGE('',*,*,#6571,.T.);
#9053=ORIENTED_EDGE('',*,*,#6689,.F.);
#9054=ORIENTED_EDGE('',*,*,#6362,.F.);
#9055=ORIENTED_EDGE('',*,*,#6688,.T.);
#9056=ORIENTED_EDGE('',*,*,#6570,.T.);
#9057=ORIENTED_EDGE('',*,*,#6690,.F.);
#9058=ORIENTED_EDGE('',*,*,#6363,.F.);
#9059=ORIENTED_EDGE('',*,*,#6689,.T.);
#9060=ORIENTED_EDGE('',*,*,#6569,.T.);
#9061=ORIENTED_EDGE('',*,*,#6691,.F.);
#9062=ORIENTED_EDGE('',*,*,#6364,.F.);
#9063=ORIENTED_EDGE('',*,*,#6690,.T.);
#9064=ORIENTED_EDGE('',*,*,#6568,.T.);
#9065=ORIENTED_EDGE('',*,*,#6692,.F.);
#9066=ORIENTED_EDGE('',*,*,#6365,.F.);
#9067=ORIENTED_EDGE('',*,*,#6691,.T.);
#9068=ORIENTED_EDGE('',*,*,#6567,.T.);
#9069=ORIENTED_EDGE('',*,*,#6693,.F.);
#9070=ORIENTED_EDGE('',*,*,#6366,.F.);
#9071=ORIENTED_EDGE('',*,*,#6692,.T.);
#9072=ORIENTED_EDGE('',*,*,#6566,.T.);
#9073=ORIENTED_EDGE('',*,*,#6694,.F.);
#9074=ORIENTED_EDGE('',*,*,#6367,.F.);
#9075=ORIENTED_EDGE('',*,*,#6693,.T.);
#9076=ORIENTED_EDGE('',*,*,#6565,.T.);
#9077=ORIENTED_EDGE('',*,*,#6695,.F.);
#9078=ORIENTED_EDGE('',*,*,#6368,.F.);
#9079=ORIENTED_EDGE('',*,*,#6694,.T.);
#9080=ORIENTED_EDGE('',*,*,#6564,.T.);
#9081=ORIENTED_EDGE('',*,*,#6696,.F.);
#9082=ORIENTED_EDGE('',*,*,#6369,.F.);
#9083=ORIENTED_EDGE('',*,*,#6695,.T.);
#9084=ORIENTED_EDGE('',*,*,#6563,.T.);
#9085=ORIENTED_EDGE('',*,*,#6697,.F.);
#9086=ORIENTED_EDGE('',*,*,#6370,.F.);
#9087=ORIENTED_EDGE('',*,*,#6696,.T.);
#9088=ORIENTED_EDGE('',*,*,#6562,.T.);
#9089=ORIENTED_EDGE('',*,*,#6698,.F.);
#9090=ORIENTED_EDGE('',*,*,#6371,.F.);
#9091=ORIENTED_EDGE('',*,*,#6697,.T.);
#9092=ORIENTED_EDGE('',*,*,#6561,.T.);
#9093=ORIENTED_EDGE('',*,*,#6699,.F.);
#9094=ORIENTED_EDGE('',*,*,#6372,.F.);
#9095=ORIENTED_EDGE('',*,*,#6698,.T.);
#9096=ORIENTED_EDGE('',*,*,#6560,.T.);
#9097=ORIENTED_EDGE('',*,*,#6700,.F.);
#9098=ORIENTED_EDGE('',*,*,#6373,.F.);
#9099=ORIENTED_EDGE('',*,*,#6699,.T.);
#9100=ORIENTED_EDGE('',*,*,#6559,.T.);
#9101=ORIENTED_EDGE('',*,*,#6701,.F.);
#9102=ORIENTED_EDGE('',*,*,#6374,.F.);
#9103=ORIENTED_EDGE('',*,*,#6700,.T.);
#9104=ORIENTED_EDGE('',*,*,#6558,.T.);
#9105=ORIENTED_EDGE('',*,*,#6702,.F.);
#9106=ORIENTED_EDGE('',*,*,#6375,.F.);
#9107=ORIENTED_EDGE('',*,*,#6701,.T.);
#9108=ORIENTED_EDGE('',*,*,#6557,.T.);
#9109=ORIENTED_EDGE('',*,*,#6703,.F.);
#9110=ORIENTED_EDGE('',*,*,#6376,.F.);
#9111=ORIENTED_EDGE('',*,*,#6702,.T.);
#9112=ORIENTED_EDGE('',*,*,#6556,.T.);
#9113=ORIENTED_EDGE('',*,*,#6704,.F.);
#9114=ORIENTED_EDGE('',*,*,#6377,.F.);
#9115=ORIENTED_EDGE('',*,*,#6703,.T.);
#9116=ORIENTED_EDGE('',*,*,#6555,.T.);
#9117=ORIENTED_EDGE('',*,*,#6705,.F.);
#9118=ORIENTED_EDGE('',*,*,#6378,.F.);
#9119=ORIENTED_EDGE('',*,*,#6704,.T.);
#9120=ORIENTED_EDGE('',*,*,#6554,.T.);
#9121=ORIENTED_EDGE('',*,*,#6706,.F.);
#9122=ORIENTED_EDGE('',*,*,#6379,.F.);
#9123=ORIENTED_EDGE('',*,*,#6705,.T.);
#9124=ORIENTED_EDGE('',*,*,#6553,.T.);
#9125=ORIENTED_EDGE('',*,*,#6707,.F.);
#9126=ORIENTED_EDGE('',*,*,#6380,.F.);
#9127=ORIENTED_EDGE('',*,*,#6706,.T.);
#9128=ORIENTED_EDGE('',*,*,#6552,.T.);
#9129=ORIENTED_EDGE('',*,*,#6708,.F.);
#9130=ORIENTED_EDGE('',*,*,#6381,.F.);
#9131=ORIENTED_EDGE('',*,*,#6707,.T.);
#9132=ORIENTED_EDGE('',*,*,#6551,.T.);
#9133=ORIENTED_EDGE('',*,*,#6709,.F.);
#9134=ORIENTED_EDGE('',*,*,#6382,.F.);
#9135=ORIENTED_EDGE('',*,*,#6708,.T.);
#9136=ORIENTED_EDGE('',*,*,#6550,.T.);
#9137=ORIENTED_EDGE('',*,*,#6710,.F.);
#9138=ORIENTED_EDGE('',*,*,#6383,.F.);
#9139=ORIENTED_EDGE('',*,*,#6709,.T.);
#9140=ORIENTED_EDGE('',*,*,#6549,.T.);
#9141=ORIENTED_EDGE('',*,*,#6711,.F.);
#9142=ORIENTED_EDGE('',*,*,#6384,.F.);
#9143=ORIENTED_EDGE('',*,*,#6710,.T.);
#9144=ORIENTED_EDGE('',*,*,#6548,.T.);
#9145=ORIENTED_EDGE('',*,*,#6712,.F.);
#9146=ORIENTED_EDGE('',*,*,#6385,.F.);
#9147=ORIENTED_EDGE('',*,*,#6711,.T.);
#9148=ORIENTED_EDGE('',*,*,#6547,.T.);
#9149=ORIENTED_EDGE('',*,*,#6713,.F.);
#9150=ORIENTED_EDGE('',*,*,#6386,.F.);
#9151=ORIENTED_EDGE('',*,*,#6712,.T.);
#9152=ORIENTED_EDGE('',*,*,#6546,.T.);
#9153=ORIENTED_EDGE('',*,*,#6714,.F.);
#9154=ORIENTED_EDGE('',*,*,#6387,.F.);
#9155=ORIENTED_EDGE('',*,*,#6713,.T.);
#9156=ORIENTED_EDGE('',*,*,#6545,.T.);
#9157=ORIENTED_EDGE('',*,*,#6715,.F.);
#9158=ORIENTED_EDGE('',*,*,#6388,.F.);
#9159=ORIENTED_EDGE('',*,*,#6714,.T.);
#9160=ORIENTED_EDGE('',*,*,#6544,.T.);
#9161=ORIENTED_EDGE('',*,*,#6716,.F.);
#9162=ORIENTED_EDGE('',*,*,#6389,.F.);
#9163=ORIENTED_EDGE('',*,*,#6715,.T.);
#9164=ORIENTED_EDGE('',*,*,#6543,.T.);
#9165=ORIENTED_EDGE('',*,*,#6717,.F.);
#9166=ORIENTED_EDGE('',*,*,#6390,.F.);
#9167=ORIENTED_EDGE('',*,*,#6716,.T.);
#9168=ORIENTED_EDGE('',*,*,#6542,.T.);
#9169=ORIENTED_EDGE('',*,*,#6718,.F.);
#9170=ORIENTED_EDGE('',*,*,#6391,.F.);
#9171=ORIENTED_EDGE('',*,*,#6717,.T.);
#9172=ORIENTED_EDGE('',*,*,#6541,.T.);
#9173=ORIENTED_EDGE('',*,*,#6719,.F.);
#9174=ORIENTED_EDGE('',*,*,#6392,.F.);
#9175=ORIENTED_EDGE('',*,*,#6718,.T.);
#9176=ORIENTED_EDGE('',*,*,#6540,.T.);
#9177=ORIENTED_EDGE('',*,*,#6720,.F.);
#9178=ORIENTED_EDGE('',*,*,#6393,.F.);
#9179=ORIENTED_EDGE('',*,*,#6719,.T.);
#9180=ORIENTED_EDGE('',*,*,#6539,.T.);
#9181=ORIENTED_EDGE('',*,*,#6721,.F.);
#9182=ORIENTED_EDGE('',*,*,#6394,.F.);
#9183=ORIENTED_EDGE('',*,*,#6720,.T.);
#9184=ORIENTED_EDGE('',*,*,#6538,.T.);
#9185=ORIENTED_EDGE('',*,*,#6722,.F.);
#9186=ORIENTED_EDGE('',*,*,#6395,.F.);
#9187=ORIENTED_EDGE('',*,*,#6721,.T.);
#9188=ORIENTED_EDGE('',*,*,#6537,.T.);
#9189=ORIENTED_EDGE('',*,*,#6723,.F.);
#9190=ORIENTED_EDGE('',*,*,#6396,.F.);
#9191=ORIENTED_EDGE('',*,*,#6722,.T.);
#9192=ORIENTED_EDGE('',*,*,#6536,.T.);
#9193=ORIENTED_EDGE('',*,*,#6724,.F.);
#9194=ORIENTED_EDGE('',*,*,#6397,.F.);
#9195=ORIENTED_EDGE('',*,*,#6723,.T.);
#9196=ORIENTED_EDGE('',*,*,#6535,.T.);
#9197=ORIENTED_EDGE('',*,*,#6725,.F.);
#9198=ORIENTED_EDGE('',*,*,#6398,.F.);
#9199=ORIENTED_EDGE('',*,*,#6724,.T.);
#9200=ORIENTED_EDGE('',*,*,#6534,.T.);
#9201=ORIENTED_EDGE('',*,*,#6726,.F.);
#9202=ORIENTED_EDGE('',*,*,#6399,.F.);
#9203=ORIENTED_EDGE('',*,*,#6725,.T.);
#9204=ORIENTED_EDGE('',*,*,#6533,.T.);
#9205=ORIENTED_EDGE('',*,*,#6727,.F.);
#9206=ORIENTED_EDGE('',*,*,#6400,.F.);
#9207=ORIENTED_EDGE('',*,*,#6726,.T.);
#9208=ORIENTED_EDGE('',*,*,#6532,.T.);
#9209=ORIENTED_EDGE('',*,*,#6728,.F.);
#9210=ORIENTED_EDGE('',*,*,#6401,.F.);
#9211=ORIENTED_EDGE('',*,*,#6727,.T.);
#9212=ORIENTED_EDGE('',*,*,#6531,.T.);
#9213=ORIENTED_EDGE('',*,*,#6729,.F.);
#9214=ORIENTED_EDGE('',*,*,#6402,.F.);
#9215=ORIENTED_EDGE('',*,*,#6728,.T.);
#9216=ORIENTED_EDGE('',*,*,#6530,.T.);
#9217=ORIENTED_EDGE('',*,*,#6730,.F.);
#9218=ORIENTED_EDGE('',*,*,#6403,.F.);
#9219=ORIENTED_EDGE('',*,*,#6729,.T.);
#9220=ORIENTED_EDGE('',*,*,#6529,.T.);
#9221=ORIENTED_EDGE('',*,*,#6731,.F.);
#9222=ORIENTED_EDGE('',*,*,#6404,.F.);
#9223=ORIENTED_EDGE('',*,*,#6730,.T.);
#9224=ORIENTED_EDGE('',*,*,#6528,.T.);
#9225=ORIENTED_EDGE('',*,*,#6732,.F.);
#9226=ORIENTED_EDGE('',*,*,#6405,.F.);
#9227=ORIENTED_EDGE('',*,*,#6731,.T.);
#9228=ORIENTED_EDGE('',*,*,#6527,.T.);
#9229=ORIENTED_EDGE('',*,*,#6733,.F.);
#9230=ORIENTED_EDGE('',*,*,#6406,.F.);
#9231=ORIENTED_EDGE('',*,*,#6732,.T.);
#9232=ORIENTED_EDGE('',*,*,#6526,.T.);
#9233=ORIENTED_EDGE('',*,*,#6734,.F.);
#9234=ORIENTED_EDGE('',*,*,#6407,.F.);
#9235=ORIENTED_EDGE('',*,*,#6733,.T.);
#9236=ORIENTED_EDGE('',*,*,#6525,.T.);
#9237=ORIENTED_EDGE('',*,*,#6735,.F.);
#9238=ORIENTED_EDGE('',*,*,#6408,.F.);
#9239=ORIENTED_EDGE('',*,*,#6734,.T.);
#9240=ORIENTED_EDGE('',*,*,#6524,.T.);
#9241=ORIENTED_EDGE('',*,*,#6736,.F.);
#9242=ORIENTED_EDGE('',*,*,#6409,.F.);
#9243=ORIENTED_EDGE('',*,*,#6735,.T.);
#9244=ORIENTED_EDGE('',*,*,#6523,.T.);
#9245=ORIENTED_EDGE('',*,*,#6737,.F.);
#9246=ORIENTED_EDGE('',*,*,#6410,.F.);
#9247=ORIENTED_EDGE('',*,*,#6736,.T.);
#9248=ORIENTED_EDGE('',*,*,#6522,.T.);
#9249=ORIENTED_EDGE('',*,*,#6738,.F.);
#9250=ORIENTED_EDGE('',*,*,#6411,.F.);
#9251=ORIENTED_EDGE('',*,*,#6737,.T.);
#9252=ORIENTED_EDGE('',*,*,#6521,.T.);
#9253=ORIENTED_EDGE('',*,*,#6739,.F.);
#9254=ORIENTED_EDGE('',*,*,#6412,.F.);
#9255=ORIENTED_EDGE('',*,*,#6738,.T.);
#9256=ORIENTED_EDGE('',*,*,#6520,.T.);
#9257=ORIENTED_EDGE('',*,*,#6740,.F.);
#9258=ORIENTED_EDGE('',*,*,#6413,.F.);
#9259=ORIENTED_EDGE('',*,*,#6739,.T.);
#9260=ORIENTED_EDGE('',*,*,#6519,.T.);
#9261=ORIENTED_EDGE('',*,*,#6741,.F.);
#9262=ORIENTED_EDGE('',*,*,#6414,.F.);
#9263=ORIENTED_EDGE('',*,*,#6740,.T.);
#9264=ORIENTED_EDGE('',*,*,#6518,.T.);
#9265=ORIENTED_EDGE('',*,*,#6742,.F.);
#9266=ORIENTED_EDGE('',*,*,#6415,.F.);
#9267=ORIENTED_EDGE('',*,*,#6741,.T.);
#9268=ORIENTED_EDGE('',*,*,#6517,.T.);
#9269=ORIENTED_EDGE('',*,*,#6743,.F.);
#9270=ORIENTED_EDGE('',*,*,#6416,.F.);
#9271=ORIENTED_EDGE('',*,*,#6742,.T.);
#9272=ORIENTED_EDGE('',*,*,#6516,.T.);
#9273=ORIENTED_EDGE('',*,*,#6744,.F.);
#9274=ORIENTED_EDGE('',*,*,#6417,.F.);
#9275=ORIENTED_EDGE('',*,*,#6743,.T.);
#9276=ORIENTED_EDGE('',*,*,#6515,.T.);
#9277=ORIENTED_EDGE('',*,*,#6745,.F.);
#9278=ORIENTED_EDGE('',*,*,#6418,.F.);
#9279=ORIENTED_EDGE('',*,*,#6744,.T.);
#9280=ORIENTED_EDGE('',*,*,#6514,.T.);
#9281=ORIENTED_EDGE('',*,*,#6746,.F.);
#9282=ORIENTED_EDGE('',*,*,#6419,.F.);
#9283=ORIENTED_EDGE('',*,*,#6745,.T.);
#9284=ORIENTED_EDGE('',*,*,#6513,.T.);
#9285=ORIENTED_EDGE('',*,*,#6747,.F.);
#9286=ORIENTED_EDGE('',*,*,#6420,.F.);
#9287=ORIENTED_EDGE('',*,*,#6746,.T.);
#9288=ORIENTED_EDGE('',*,*,#6512,.T.);
#9289=ORIENTED_EDGE('',*,*,#6748,.F.);
#9290=ORIENTED_EDGE('',*,*,#6421,.F.);
#9291=ORIENTED_EDGE('',*,*,#6747,.T.);
#9292=ORIENTED_EDGE('',*,*,#6511,.T.);
#9293=ORIENTED_EDGE('',*,*,#6749,.F.);
#9294=ORIENTED_EDGE('',*,*,#6422,.F.);
#9295=ORIENTED_EDGE('',*,*,#6748,.T.);
#9296=ORIENTED_EDGE('',*,*,#6510,.T.);
#9297=ORIENTED_EDGE('',*,*,#6750,.F.);
#9298=ORIENTED_EDGE('',*,*,#6423,.F.);
#9299=ORIENTED_EDGE('',*,*,#6749,.T.);
#9300=ORIENTED_EDGE('',*,*,#6509,.T.);
#9301=ORIENTED_EDGE('',*,*,#6751,.F.);
#9302=ORIENTED_EDGE('',*,*,#6424,.F.);
#9303=ORIENTED_EDGE('',*,*,#6750,.T.);
#9304=ORIENTED_EDGE('',*,*,#6508,.T.);
#9305=ORIENTED_EDGE('',*,*,#6752,.F.);
#9306=ORIENTED_EDGE('',*,*,#6425,.F.);
#9307=ORIENTED_EDGE('',*,*,#6751,.T.);
#9308=ORIENTED_EDGE('',*,*,#6507,.T.);
#9309=ORIENTED_EDGE('',*,*,#6753,.F.);
#9310=ORIENTED_EDGE('',*,*,#6426,.F.);
#9311=ORIENTED_EDGE('',*,*,#6752,.T.);
#9312=ORIENTED_EDGE('',*,*,#6506,.T.);
#9313=ORIENTED_EDGE('',*,*,#6754,.F.);
#9314=ORIENTED_EDGE('',*,*,#6427,.F.);
#9315=ORIENTED_EDGE('',*,*,#6753,.T.);
#9316=ORIENTED_EDGE('',*,*,#6505,.T.);
#9317=ORIENTED_EDGE('',*,*,#6755,.F.);
#9318=ORIENTED_EDGE('',*,*,#6428,.F.);
#9319=ORIENTED_EDGE('',*,*,#6754,.T.);
#9320=ORIENTED_EDGE('',*,*,#6504,.T.);
#9321=ORIENTED_EDGE('',*,*,#6756,.F.);
#9322=ORIENTED_EDGE('',*,*,#6429,.F.);
#9323=ORIENTED_EDGE('',*,*,#6755,.T.);
#9324=ORIENTED_EDGE('',*,*,#6503,.T.);
#9325=ORIENTED_EDGE('',*,*,#6757,.F.);
#9326=ORIENTED_EDGE('',*,*,#6430,.F.);
#9327=ORIENTED_EDGE('',*,*,#6756,.T.);
#9328=ORIENTED_EDGE('',*,*,#6502,.T.);
#9329=ORIENTED_EDGE('',*,*,#6758,.F.);
#9330=ORIENTED_EDGE('',*,*,#6431,.F.);
#9331=ORIENTED_EDGE('',*,*,#6757,.T.);
#9332=ORIENTED_EDGE('',*,*,#6501,.T.);
#9333=ORIENTED_EDGE('',*,*,#6759,.F.);
#9334=ORIENTED_EDGE('',*,*,#6432,.F.);
#9335=ORIENTED_EDGE('',*,*,#6758,.T.);
#9336=ORIENTED_EDGE('',*,*,#6500,.T.);
#9337=ORIENTED_EDGE('',*,*,#6760,.F.);
#9338=ORIENTED_EDGE('',*,*,#6433,.F.);
#9339=ORIENTED_EDGE('',*,*,#6759,.T.);
#9340=ORIENTED_EDGE('',*,*,#6499,.T.);
#9341=ORIENTED_EDGE('',*,*,#6761,.F.);
#9342=ORIENTED_EDGE('',*,*,#6434,.F.);
#9343=ORIENTED_EDGE('',*,*,#6760,.T.);
#9344=ORIENTED_EDGE('',*,*,#6498,.T.);
#9345=ORIENTED_EDGE('',*,*,#6762,.F.);
#9346=ORIENTED_EDGE('',*,*,#6435,.F.);
#9347=ORIENTED_EDGE('',*,*,#6761,.T.);
#9348=ORIENTED_EDGE('',*,*,#6497,.T.);
#9349=ORIENTED_EDGE('',*,*,#6763,.F.);
#9350=ORIENTED_EDGE('',*,*,#6436,.F.);
#9351=ORIENTED_EDGE('',*,*,#6762,.T.);
#9352=ORIENTED_EDGE('',*,*,#6496,.T.);
#9353=ORIENTED_EDGE('',*,*,#6764,.F.);
#9354=ORIENTED_EDGE('',*,*,#6437,.F.);
#9355=ORIENTED_EDGE('',*,*,#6763,.T.);
#9356=ORIENTED_EDGE('',*,*,#6495,.T.);
#9357=ORIENTED_EDGE('',*,*,#6765,.F.);
#9358=ORIENTED_EDGE('',*,*,#6438,.F.);
#9359=ORIENTED_EDGE('',*,*,#6764,.T.);
#9360=ORIENTED_EDGE('',*,*,#6494,.T.);
#9361=ORIENTED_EDGE('',*,*,#6766,.F.);
#9362=ORIENTED_EDGE('',*,*,#6439,.F.);
#9363=ORIENTED_EDGE('',*,*,#6765,.T.);
#9364=ORIENTED_EDGE('',*,*,#6493,.T.);
#9365=ORIENTED_EDGE('',*,*,#6767,.F.);
#9366=ORIENTED_EDGE('',*,*,#6440,.F.);
#9367=ORIENTED_EDGE('',*,*,#6766,.T.);
#9368=ORIENTED_EDGE('',*,*,#6492,.T.);
#9369=ORIENTED_EDGE('',*,*,#6768,.F.);
#9370=ORIENTED_EDGE('',*,*,#6441,.F.);
#9371=ORIENTED_EDGE('',*,*,#6767,.T.);
#9372=ORIENTED_EDGE('',*,*,#6491,.T.);
#9373=ORIENTED_EDGE('',*,*,#6654,.F.);
#9374=ORIENTED_EDGE('',*,*,#6442,.F.);
#9375=ORIENTED_EDGE('',*,*,#6768,.T.);
#9376=ORIENTED_EDGE('',*,*,#6606,.F.);
#9377=ORIENTED_EDGE('',*,*,#6769,.F.);
#9378=ORIENTED_EDGE('',*,*,#6444,.T.);
#9379=ORIENTED_EDGE('',*,*,#6770,.T.);
#9380=ORIENTED_EDGE('',*,*,#6607,.F.);
#9381=ORIENTED_EDGE('',*,*,#6770,.F.);
#9382=ORIENTED_EDGE('',*,*,#6443,.T.);
#9383=ORIENTED_EDGE('',*,*,#6771,.T.);
#9384=ORIENTED_EDGE('',*,*,#6608,.F.);
#9385=ORIENTED_EDGE('',*,*,#6771,.F.);
#9386=ORIENTED_EDGE('',*,*,#6450,.T.);
#9387=ORIENTED_EDGE('',*,*,#6772,.T.);
#9388=ORIENTED_EDGE('',*,*,#6609,.F.);
#9389=ORIENTED_EDGE('',*,*,#6772,.F.);
#9390=ORIENTED_EDGE('',*,*,#6449,.T.);
#9391=ORIENTED_EDGE('',*,*,#6773,.T.);
#9392=ORIENTED_EDGE('',*,*,#6610,.F.);
#9393=ORIENTED_EDGE('',*,*,#6773,.F.);
#9394=ORIENTED_EDGE('',*,*,#6448,.T.);
#9395=ORIENTED_EDGE('',*,*,#6774,.T.);
#9396=ORIENTED_EDGE('',*,*,#6611,.F.);
#9397=ORIENTED_EDGE('',*,*,#6774,.F.);
#9398=ORIENTED_EDGE('',*,*,#6447,.T.);
#9399=ORIENTED_EDGE('',*,*,#6775,.T.);
#9400=ORIENTED_EDGE('',*,*,#6612,.F.);
#9401=ORIENTED_EDGE('',*,*,#6775,.F.);
#9402=ORIENTED_EDGE('',*,*,#6446,.T.);
#9403=ORIENTED_EDGE('',*,*,#6776,.T.);
#9404=ORIENTED_EDGE('',*,*,#6613,.F.);
#9405=ORIENTED_EDGE('',*,*,#6776,.F.);
#9406=ORIENTED_EDGE('',*,*,#6445,.T.);
#9407=ORIENTED_EDGE('',*,*,#6769,.T.);
#9408=ORIENTED_EDGE('',*,*,#6638,.F.);
#9409=ORIENTED_EDGE('',*,*,#6777,.F.);
#9410=ORIENTED_EDGE('',*,*,#6452,.T.);
#9411=ORIENTED_EDGE('',*,*,#6778,.T.);
#9412=ORIENTED_EDGE('',*,*,#6639,.F.);
#9413=ORIENTED_EDGE('',*,*,#6778,.F.);
#9414=ORIENTED_EDGE('',*,*,#6451,.T.);
#9415=ORIENTED_EDGE('',*,*,#6779,.T.);
#9416=ORIENTED_EDGE('',*,*,#6640,.F.);
#9417=ORIENTED_EDGE('',*,*,#6779,.F.);
#9418=ORIENTED_EDGE('',*,*,#6465,.T.);
#9419=ORIENTED_EDGE('',*,*,#6780,.T.);
#9420=ORIENTED_EDGE('',*,*,#6641,.F.);
#9421=ORIENTED_EDGE('',*,*,#6780,.F.);
#9422=ORIENTED_EDGE('',*,*,#6464,.T.);
#9423=ORIENTED_EDGE('',*,*,#6326,.T.);
#9424=ORIENTED_EDGE('',*,*,#6642,.F.);
#9425=ORIENTED_EDGE('',*,*,#6324,.F.);
#9426=ORIENTED_EDGE('',*,*,#6463,.T.);
#9427=ORIENTED_EDGE('',*,*,#6781,.T.);
#9428=ORIENTED_EDGE('',*,*,#6643,.F.);
#9429=ORIENTED_EDGE('',*,*,#6781,.F.);
#9430=ORIENTED_EDGE('',*,*,#6462,.T.);
#9431=ORIENTED_EDGE('',*,*,#6782,.T.);
#9432=ORIENTED_EDGE('',*,*,#6644,.F.);
#9433=ORIENTED_EDGE('',*,*,#6782,.F.);
#9434=ORIENTED_EDGE('',*,*,#6461,.T.);
#9435=ORIENTED_EDGE('',*,*,#6783,.T.);
#9436=ORIENTED_EDGE('',*,*,#6645,.F.);
#9437=ORIENTED_EDGE('',*,*,#6783,.F.);
#9438=ORIENTED_EDGE('',*,*,#6460,.T.);
#9439=ORIENTED_EDGE('',*,*,#6784,.T.);
#9440=ORIENTED_EDGE('',*,*,#6646,.F.);
#9441=ORIENTED_EDGE('',*,*,#6784,.F.);
#9442=ORIENTED_EDGE('',*,*,#6459,.T.);
#9443=ORIENTED_EDGE('',*,*,#6785,.T.);
#9444=ORIENTED_EDGE('',*,*,#6647,.F.);
#9445=ORIENTED_EDGE('',*,*,#6785,.F.);
#9446=ORIENTED_EDGE('',*,*,#6458,.T.);
#9447=ORIENTED_EDGE('',*,*,#6786,.T.);
#9448=ORIENTED_EDGE('',*,*,#6648,.F.);
#9449=ORIENTED_EDGE('',*,*,#6786,.F.);
#9450=ORIENTED_EDGE('',*,*,#6457,.T.);
#9451=ORIENTED_EDGE('',*,*,#6787,.T.);
#9452=ORIENTED_EDGE('',*,*,#6649,.F.);
#9453=ORIENTED_EDGE('',*,*,#6787,.F.);
#9454=ORIENTED_EDGE('',*,*,#6456,.T.);
#9455=ORIENTED_EDGE('',*,*,#6788,.T.);
#9456=ORIENTED_EDGE('',*,*,#6650,.F.);
#9457=ORIENTED_EDGE('',*,*,#6788,.F.);
#9458=ORIENTED_EDGE('',*,*,#6455,.T.);
#9459=ORIENTED_EDGE('',*,*,#6789,.T.);
#9460=ORIENTED_EDGE('',*,*,#6651,.F.);
#9461=ORIENTED_EDGE('',*,*,#6789,.F.);
#9462=ORIENTED_EDGE('',*,*,#6454,.T.);
#9463=ORIENTED_EDGE('',*,*,#6790,.T.);
#9464=ORIENTED_EDGE('',*,*,#6652,.F.);
#9465=ORIENTED_EDGE('',*,*,#6790,.F.);
#9466=ORIENTED_EDGE('',*,*,#6453,.T.);
#9467=ORIENTED_EDGE('',*,*,#6777,.T.);
#9468=ORIENTED_EDGE('',*,*,#6614,.F.);
#9469=ORIENTED_EDGE('',*,*,#6791,.F.);
#9470=ORIENTED_EDGE('',*,*,#6467,.T.);
#9471=ORIENTED_EDGE('',*,*,#6792,.T.);
#9472=ORIENTED_EDGE('',*,*,#6615,.F.);
#9473=ORIENTED_EDGE('',*,*,#6792,.F.);
#9474=ORIENTED_EDGE('',*,*,#6466,.T.);
#9475=ORIENTED_EDGE('',*,*,#6793,.T.);
#9476=ORIENTED_EDGE('',*,*,#6616,.F.);
#9477=ORIENTED_EDGE('',*,*,#6793,.F.);
#9478=ORIENTED_EDGE('',*,*,#6473,.T.);
#9479=ORIENTED_EDGE('',*,*,#6794,.T.);
#9480=ORIENTED_EDGE('',*,*,#6617,.F.);
#9481=ORIENTED_EDGE('',*,*,#6794,.F.);
#9482=ORIENTED_EDGE('',*,*,#6472,.T.);
#9483=ORIENTED_EDGE('',*,*,#6795,.T.);
#9484=ORIENTED_EDGE('',*,*,#6618,.F.);
#9485=ORIENTED_EDGE('',*,*,#6795,.F.);
#9486=ORIENTED_EDGE('',*,*,#6471,.T.);
#9487=ORIENTED_EDGE('',*,*,#6796,.T.);
#9488=ORIENTED_EDGE('',*,*,#6619,.F.);
#9489=ORIENTED_EDGE('',*,*,#6796,.F.);
#9490=ORIENTED_EDGE('',*,*,#6470,.T.);
#9491=ORIENTED_EDGE('',*,*,#6797,.T.);
#9492=ORIENTED_EDGE('',*,*,#6620,.F.);
#9493=ORIENTED_EDGE('',*,*,#6797,.F.);
#9494=ORIENTED_EDGE('',*,*,#6469,.T.);
#9495=ORIENTED_EDGE('',*,*,#6798,.T.);
#9496=ORIENTED_EDGE('',*,*,#6621,.F.);
#9497=ORIENTED_EDGE('',*,*,#6798,.F.);
#9498=ORIENTED_EDGE('',*,*,#6468,.T.);
#9499=ORIENTED_EDGE('',*,*,#6791,.T.);
#9500=ORIENTED_EDGE('',*,*,#6630,.F.);
#9501=ORIENTED_EDGE('',*,*,#6799,.F.);
#9502=ORIENTED_EDGE('',*,*,#6475,.T.);
#9503=ORIENTED_EDGE('',*,*,#6800,.T.);
#9504=ORIENTED_EDGE('',*,*,#6631,.F.);
#9505=ORIENTED_EDGE('',*,*,#6800,.F.);
#9506=ORIENTED_EDGE('',*,*,#6474,.T.);
#9507=ORIENTED_EDGE('',*,*,#6801,.T.);
#9508=ORIENTED_EDGE('',*,*,#6632,.F.);
#9509=ORIENTED_EDGE('',*,*,#6801,.F.);
#9510=ORIENTED_EDGE('',*,*,#6481,.T.);
#9511=ORIENTED_EDGE('',*,*,#6802,.T.);
#9512=ORIENTED_EDGE('',*,*,#6633,.F.);
#9513=ORIENTED_EDGE('',*,*,#6802,.F.);
#9514=ORIENTED_EDGE('',*,*,#6480,.T.);
#9515=ORIENTED_EDGE('',*,*,#6803,.T.);
#9516=ORIENTED_EDGE('',*,*,#6634,.F.);
#9517=ORIENTED_EDGE('',*,*,#6803,.F.);
#9518=ORIENTED_EDGE('',*,*,#6479,.T.);
#9519=ORIENTED_EDGE('',*,*,#6804,.T.);
#9520=ORIENTED_EDGE('',*,*,#6635,.F.);
#9521=ORIENTED_EDGE('',*,*,#6804,.F.);
#9522=ORIENTED_EDGE('',*,*,#6478,.T.);
#9523=ORIENTED_EDGE('',*,*,#6805,.T.);
#9524=ORIENTED_EDGE('',*,*,#6636,.F.);
#9525=ORIENTED_EDGE('',*,*,#6805,.F.);
#9526=ORIENTED_EDGE('',*,*,#6477,.T.);
#9527=ORIENTED_EDGE('',*,*,#6806,.T.);
#9528=ORIENTED_EDGE('',*,*,#6637,.F.);
#9529=ORIENTED_EDGE('',*,*,#6806,.F.);
#9530=ORIENTED_EDGE('',*,*,#6476,.T.);
#9531=ORIENTED_EDGE('',*,*,#6799,.T.);
#9532=ORIENTED_EDGE('',*,*,#6622,.F.);
#9533=ORIENTED_EDGE('',*,*,#6807,.F.);
#9534=ORIENTED_EDGE('',*,*,#6483,.T.);
#9535=ORIENTED_EDGE('',*,*,#6808,.T.);
#9536=ORIENTED_EDGE('',*,*,#6623,.F.);
#9537=ORIENTED_EDGE('',*,*,#6808,.F.);
#9538=ORIENTED_EDGE('',*,*,#6482,.T.);
#9539=ORIENTED_EDGE('',*,*,#6809,.T.);
#9540=ORIENTED_EDGE('',*,*,#6624,.F.);
#9541=ORIENTED_EDGE('',*,*,#6809,.F.);
#9542=ORIENTED_EDGE('',*,*,#6489,.T.);
#9543=ORIENTED_EDGE('',*,*,#6810,.T.);
#9544=ORIENTED_EDGE('',*,*,#6625,.F.);
#9545=ORIENTED_EDGE('',*,*,#6810,.F.);
#9546=ORIENTED_EDGE('',*,*,#6488,.T.);
#9547=ORIENTED_EDGE('',*,*,#6811,.T.);
#9548=ORIENTED_EDGE('',*,*,#6626,.F.);
#9549=ORIENTED_EDGE('',*,*,#6811,.F.);
#9550=ORIENTED_EDGE('',*,*,#6487,.T.);
#9551=ORIENTED_EDGE('',*,*,#6812,.T.);
#9552=ORIENTED_EDGE('',*,*,#6627,.F.);
#9553=ORIENTED_EDGE('',*,*,#6812,.F.);
#9554=ORIENTED_EDGE('',*,*,#6486,.T.);
#9555=ORIENTED_EDGE('',*,*,#6813,.T.);
#9556=ORIENTED_EDGE('',*,*,#6628,.F.);
#9557=ORIENTED_EDGE('',*,*,#6813,.F.);
#9558=ORIENTED_EDGE('',*,*,#6485,.T.);
#9559=ORIENTED_EDGE('',*,*,#6814,.T.);
#9560=ORIENTED_EDGE('',*,*,#6629,.F.);
#9561=ORIENTED_EDGE('',*,*,#6814,.F.);
#9562=ORIENTED_EDGE('',*,*,#6484,.T.);
#9563=ORIENTED_EDGE('',*,*,#6807,.T.);
#10253=CYLINDRICAL_SURFACE('',#11713,3.65);
#10254=CYLINDRICAL_SURFACE('',#11857,0.200000403400263);
#10255=CYLINDRICAL_SURFACE('',#11859,0.600000196920858);
#10256=CYLINDRICAL_SURFACE('',#11861,0.200000373597978);
#10257=CYLINDRICAL_SURFACE('',#11863,0.199999419924102);
#10258=CYLINDRICAL_SURFACE('',#11865,0.20000038104856);
#10259=CYLINDRICAL_SURFACE('',#11867,1.99999965375783);
#10260=CYLINDRICAL_SURFACE('',#11869,0.200000284191204);
#10261=CYLINDRICAL_SURFACE('',#11871,0.200000284191204);
#10262=CYLINDRICAL_SURFACE('',#11873,0.200000284191218);
#10263=CYLINDRICAL_SURFACE('',#11875,0.60000037573478);
#10264=CYLINDRICAL_SURFACE('',#11877,0.200000284191204);
#10265=CYLINDRICAL_SURFACE('',#11886,0.20000028419119);
#10266=CYLINDRICAL_SURFACE('',#11888,0.60000037573478);
#10267=CYLINDRICAL_SURFACE('',#11890,0.200000284191218);
#10268=CYLINDRICAL_SURFACE('',#11892,0.200000284191204);
#10269=CYLINDRICAL_SURFACE('',#11894,0.200000284191218);
#10270=CYLINDRICAL_SURFACE('',#11896,1.99999965375781);
#10271=CYLINDRICAL_SURFACE('',#11898,0.200000381048546);
#10272=CYLINDRICAL_SURFACE('',#11900,0.199999419924102);
#10273=CYLINDRICAL_SURFACE('',#11902,0.200000373597978);
#10274=CYLINDRICAL_SURFACE('',#11904,0.600000196920858);
#10275=CYLINDRICAL_SURFACE('',#11906,0.200000403400263);
#10276=CYLINDRICAL_SURFACE('',#11915,0.200000403400263);
#10277=CYLINDRICAL_SURFACE('',#11917,0.600000196920858);
#10278=CYLINDRICAL_SURFACE('',#11919,0.200000373597978);
#10279=CYLINDRICAL_SURFACE('',#11921,0.199999419924102);
#10280=CYLINDRICAL_SURFACE('',#11923,0.200000381048546);
#10281=CYLINDRICAL_SURFACE('',#11925,1.99999965375781);
#10282=CYLINDRICAL_SURFACE('',#11927,0.200000284191204);
#10283=CYLINDRICAL_SURFACE('',#11929,0.200000284191204);
#10284=CYLINDRICAL_SURFACE('',#11931,0.200000284191218);
#10285=CYLINDRICAL_SURFACE('',#11933,0.600000375734794);
#10286=CYLINDRICAL_SURFACE('',#11935,0.200000284191204);
#10287=CYLINDRICAL_SURFACE('',#11944,0.200000284191204);
#10288=CYLINDRICAL_SURFACE('',#11946,0.60000037573478);
#10289=CYLINDRICAL_SURFACE('',#11948,0.200000284191218);
#10290=CYLINDRICAL_SURFACE('',#11950,0.20000028419119);
#10291=CYLINDRICAL_SURFACE('',#11952,0.200000284191218);
#10292=CYLINDRICAL_SURFACE('',#11954,1.9999996537578);
#10293=CYLINDRICAL_SURFACE('',#11956,0.200000381048532);
#10294=CYLINDRICAL_SURFACE('',#11958,0.199999419924102);
#10295=CYLINDRICAL_SURFACE('',#11960,0.200000373597992);
#10296=CYLINDRICAL_SURFACE('',#11962,0.600000196920844);
#10297=CYLINDRICAL_SURFACE('',#11964,0.200000403400263);
#10298=CYLINDRICAL_SURFACE('',#11968,0.999999990441758);
#10299=CYLINDRICAL_SURFACE('',#11970,0.999999990441772);
#10300=CYLINDRICAL_SURFACE('',#11972,0.999999990441772);
#10301=CYLINDRICAL_SURFACE('',#11974,0.999999990441758);
#10302=CYLINDRICAL_SURFACE('',#11976,3.65);
#10303=CYLINDRICAL_SURFACE('',#11978,5.50000000000001);
#10304=CYLINDRICAL_SURFACE('',#11981,5.50000000000001);
#10305=CYLINDRICAL_SURFACE('',#11983,3.65);
#10306=CYLINDRICAL_SURFACE('',#11985,5.50000000000001);
#10307=CYLINDRICAL_SURFACE('',#11987,3.65);
#10308=CYLINDRICAL_SURFACE('',#11989,5.50000000000001);
#10309=CYLINDRICAL_SURFACE('',#11991,0.999999990441758);
#10310=CYLINDRICAL_SURFACE('',#11993,0.999999990441758);
#10311=CYLINDRICAL_SURFACE('',#11995,0.999999990441758);
#10312=CYLINDRICAL_SURFACE('',#11997,0.999999990441758);
#10313=CYLINDRICAL_SURFACE('',#11999,0.999999990441758);
#10314=CYLINDRICAL_SURFACE('',#12001,0.999999990441758);
#10315=CYLINDRICAL_SURFACE('',#12003,0.999999990441772);
#10316=CYLINDRICAL_SURFACE('',#12005,0.999999990441772);
#10317=CYLINDRICAL_SURFACE('',#12007,0.999999990441758);
#10318=CYLINDRICAL_SURFACE('',#12009,0.999999990441758);
#10319=CYLINDRICAL_SURFACE('',#12011,0.999999990441758);
#10320=CYLINDRICAL_SURFACE('',#12013,0.999999990441758);
#10663=ADVANCED_FACE('',(#1026),#10253,.F.);
#10664=ADVANCED_FACE('',(#1027,#346,#347,#348,#349,#350),#568,.T.);
#10665=ADVANCED_FACE('',(#1028,#351,#352,#353,#354,#355),#569,.F.);
#10666=ADVANCED_FACE('',(#1029),#570,.F.);
#10667=ADVANCED_FACE('',(#1030),#571,.F.);
#10668=ADVANCED_FACE('',(#1031),#572,.F.);
#10669=ADVANCED_FACE('',(#1032),#573,.F.);
#10670=ADVANCED_FACE('',(#1033),#574,.F.);
#10671=ADVANCED_FACE('',(#1034),#10254,.F.);
#10672=ADVANCED_FACE('',(#1035),#575,.F.);
#10673=ADVANCED_FACE('',(#1036),#10255,.T.);
#10674=ADVANCED_FACE('',(#1037),#576,.F.);
#10675=ADVANCED_FACE('',(#1038),#10256,.T.);
#10676=ADVANCED_FACE('',(#1039),#577,.F.);
#10677=ADVANCED_FACE('',(#1040),#10257,.F.);
#10678=ADVANCED_FACE('',(#1041),#578,.F.);
#10679=ADVANCED_FACE('',(#1042),#10258,.T.);
#10680=ADVANCED_FACE('',(#1043),#579,.F.);
#10681=ADVANCED_FACE('',(#1044),#10259,.T.);
#10682=ADVANCED_FACE('',(#1045),#580,.F.);
#10683=ADVANCED_FACE('',(#1046),#10260,.T.);
#10684=ADVANCED_FACE('',(#1047),#581,.F.);
#10685=ADVANCED_FACE('',(#1048),#10261,.F.);
#10686=ADVANCED_FACE('',(#1049),#582,.F.);
#10687=ADVANCED_FACE('',(#1050),#10262,.T.);
#10688=ADVANCED_FACE('',(#1051),#583,.F.);
#10689=ADVANCED_FACE('',(#1052),#10263,.T.);
#10690=ADVANCED_FACE('',(#1053),#584,.F.);
#10691=ADVANCED_FACE('',(#1054),#10264,.F.);
#10692=ADVANCED_FACE('',(#1055),#585,.F.);
#10693=ADVANCED_FACE('',(#1056),#586,.F.);
#10694=ADVANCED_FACE('',(#1057),#587,.F.);
#10695=ADVANCED_FACE('',(#1058),#588,.F.);
#10696=ADVANCED_FACE('',(#1059),#589,.F.);
#10697=ADVANCED_FACE('',(#1060),#590,.F.);
#10698=ADVANCED_FACE('',(#1061),#591,.F.);
#10699=ADVANCED_FACE('',(#1062),#592,.F.);
#10700=ADVANCED_FACE('',(#1063),#10265,.F.);
#10701=ADVANCED_FACE('',(#1064),#593,.F.);
#10702=ADVANCED_FACE('',(#1065),#10266,.T.);
#10703=ADVANCED_FACE('',(#1066),#594,.F.);
#10704=ADVANCED_FACE('',(#1067),#10267,.T.);
#10705=ADVANCED_FACE('',(#1068),#595,.F.);
#10706=ADVANCED_FACE('',(#1069),#10268,.F.);
#10707=ADVANCED_FACE('',(#1070),#596,.F.);
#10708=ADVANCED_FACE('',(#1071),#10269,.T.);
#10709=ADVANCED_FACE('',(#1072),#597,.F.);
#10710=ADVANCED_FACE('',(#1073),#10270,.T.);
#10711=ADVANCED_FACE('',(#1074),#598,.F.);
#10712=ADVANCED_FACE('',(#1075),#10271,.T.);
#10713=ADVANCED_FACE('',(#1076),#599,.F.);
#10714=ADVANCED_FACE('',(#1077),#10272,.F.);
#10715=ADVANCED_FACE('',(#1078),#600,.F.);
#10716=ADVANCED_FACE('',(#1079),#10273,.T.);
#10717=ADVANCED_FACE('',(#1080),#601,.F.);
#10718=ADVANCED_FACE('',(#1081),#10274,.T.);
#10719=ADVANCED_FACE('',(#1082),#602,.F.);
#10720=ADVANCED_FACE('',(#1083),#10275,.F.);
#10721=ADVANCED_FACE('',(#1084),#603,.F.);
#10722=ADVANCED_FACE('',(#1085),#604,.F.);
#10723=ADVANCED_FACE('',(#1086),#605,.F.);
#10724=ADVANCED_FACE('',(#1087),#606,.F.);
#10725=ADVANCED_FACE('',(#1088),#607,.F.);
#10726=ADVANCED_FACE('',(#1089),#608,.F.);
#10727=ADVANCED_FACE('',(#1090),#609,.F.);
#10728=ADVANCED_FACE('',(#1091),#610,.F.);
#10729=ADVANCED_FACE('',(#1092),#10276,.F.);
#10730=ADVANCED_FACE('',(#1093),#611,.F.);
#10731=ADVANCED_FACE('',(#1094),#10277,.T.);
#10732=ADVANCED_FACE('',(#1095),#612,.F.);
#10733=ADVANCED_FACE('',(#1096),#10278,.T.);
#10734=ADVANCED_FACE('',(#1097),#613,.F.);
#10735=ADVANCED_FACE('',(#1098),#10279,.F.);
#10736=ADVANCED_FACE('',(#1099),#614,.F.);
#10737=ADVANCED_FACE('',(#1100),#10280,.T.);
#10738=ADVANCED_FACE('',(#1101),#615,.F.);
#10739=ADVANCED_FACE('',(#1102),#10281,.T.);
#10740=ADVANCED_FACE('',(#1103),#616,.F.);
#10741=ADVANCED_FACE('',(#1104),#10282,.T.);
#10742=ADVANCED_FACE('',(#1105),#617,.F.);
#10743=ADVANCED_FACE('',(#1106),#10283,.F.);
#10744=ADVANCED_FACE('',(#1107),#618,.F.);
#10745=ADVANCED_FACE('',(#1108),#10284,.T.);
#10746=ADVANCED_FACE('',(#1109),#619,.F.);
#10747=ADVANCED_FACE('',(#1110),#10285,.T.);
#10748=ADVANCED_FACE('',(#1111),#620,.F.);
#10749=ADVANCED_FACE('',(#1112),#10286,.F.);
#10750=ADVANCED_FACE('',(#1113),#621,.F.);
#10751=ADVANCED_FACE('',(#1114),#622,.F.);
#10752=ADVANCED_FACE('',(#1115),#623,.F.);
#10753=ADVANCED_FACE('',(#1116),#624,.F.);
#10754=ADVANCED_FACE('',(#1117),#625,.F.);
#10755=ADVANCED_FACE('',(#1118),#626,.F.);
#10756=ADVANCED_FACE('',(#1119),#627,.F.);
#10757=ADVANCED_FACE('',(#1120),#628,.F.);
#10758=ADVANCED_FACE('',(#1121),#10287,.F.);
#10759=ADVANCED_FACE('',(#1122),#629,.F.);
#10760=ADVANCED_FACE('',(#1123),#10288,.T.);
#10761=ADVANCED_FACE('',(#1124),#630,.F.);
#10762=ADVANCED_FACE('',(#1125),#10289,.T.);
#10763=ADVANCED_FACE('',(#1126),#631,.F.);
#10764=ADVANCED_FACE('',(#1127),#10290,.F.);
#10765=ADVANCED_FACE('',(#1128),#632,.F.);
#10766=ADVANCED_FACE('',(#1129),#10291,.T.);
#10767=ADVANCED_FACE('',(#1130),#633,.F.);
#10768=ADVANCED_FACE('',(#1131),#10292,.T.);
#10769=ADVANCED_FACE('',(#1132),#634,.F.);
#10770=ADVANCED_FACE('',(#1133),#10293,.T.);
#10771=ADVANCED_FACE('',(#1134),#635,.F.);
#10772=ADVANCED_FACE('',(#1135),#10294,.F.);
#10773=ADVANCED_FACE('',(#1136),#636,.F.);
#10774=ADVANCED_FACE('',(#1137),#10295,.T.);
#10775=ADVANCED_FACE('',(#1138),#637,.F.);
#10776=ADVANCED_FACE('',(#1139),#10296,.T.);
#10777=ADVANCED_FACE('',(#1140),#638,.F.);
#10778=ADVANCED_FACE('',(#1141),#10297,.F.);
#10779=ADVANCED_FACE('',(#1142),#639,.F.);
#10780=ADVANCED_FACE('',(#1143),#640,.F.);
#10781=ADVANCED_FACE('',(#1144),#641,.F.);
#10782=ADVANCED_FACE('',(#1145),#10298,.F.);
#10783=ADVANCED_FACE('',(#1146),#642,.T.);
#10784=ADVANCED_FACE('',(#1147),#10299,.F.);
#10785=ADVANCED_FACE('',(#1148),#643,.T.);
#10786=ADVANCED_FACE('',(#1149),#10300,.F.);
#10787=ADVANCED_FACE('',(#1150),#644,.T.);
#10788=ADVANCED_FACE('',(#1151),#10301,.F.);
#10789=ADVANCED_FACE('',(#1152),#645,.T.);
#10790=ADVANCED_FACE('',(#1153),#10302,.F.);
#10791=ADVANCED_FACE('',(#1154),#646,.T.);
#10792=ADVANCED_FACE('',(#1155),#10303,.F.);
#10793=ADVANCED_FACE('',(#1156),#647,.T.);
#10794=ADVANCED_FACE('',(#1157),#648,.T.);
#10795=ADVANCED_FACE('',(#1158),#10304,.F.);
#10796=ADVANCED_FACE('',(#1159),#649,.T.);
#10797=ADVANCED_FACE('',(#1160),#10305,.F.);
#10798=ADVANCED_FACE('',(#1161),#650,.T.);
#10799=ADVANCED_FACE('',(#1162),#10306,.F.);
#10800=ADVANCED_FACE('',(#1163),#651,.T.);
#10801=ADVANCED_FACE('',(#1164),#10307,.F.);
#10802=ADVANCED_FACE('',(#1165),#652,.T.);
#10803=ADVANCED_FACE('',(#1166),#10308,.F.);
#10804=ADVANCED_FACE('',(#1167),#653,.T.);
#10805=ADVANCED_FACE('',(#1168),#10309,.F.);
#10806=ADVANCED_FACE('',(#1169),#654,.T.);
#10807=ADVANCED_FACE('',(#1170),#10310,.F.);
#10808=ADVANCED_FACE('',(#1171),#655,.T.);
#10809=ADVANCED_FACE('',(#1172),#10311,.F.);
#10810=ADVANCED_FACE('',(#1173),#656,.T.);
#10811=ADVANCED_FACE('',(#1174),#10312,.F.);
#10812=ADVANCED_FACE('',(#1175),#657,.T.);
#10813=ADVANCED_FACE('',(#1176),#10313,.F.);
#10814=ADVANCED_FACE('',(#1177),#658,.T.);
#10815=ADVANCED_FACE('',(#1178),#10314,.F.);
#10816=ADVANCED_FACE('',(#1179),#659,.T.);
#10817=ADVANCED_FACE('',(#1180),#10315,.F.);
#10818=ADVANCED_FACE('',(#1181),#660,.T.);
#10819=ADVANCED_FACE('',(#1182),#10316,.F.);
#10820=ADVANCED_FACE('',(#1183),#661,.T.);
#10821=ADVANCED_FACE('',(#1184),#10317,.F.);
#10822=ADVANCED_FACE('',(#1185),#662,.T.);
#10823=ADVANCED_FACE('',(#1186),#10318,.F.);
#10824=ADVANCED_FACE('',(#1187),#663,.T.);
#10825=ADVANCED_FACE('',(#1188),#10319,.F.);
#10826=ADVANCED_FACE('',(#1189),#664,.T.);
#10827=ADVANCED_FACE('',(#1190),#10320,.F.);
#10828=ADVANCED_FACE('',(#1191),#665,.T.);
#10968=CLOSED_SHELL('',(#10663,#10664,#10665,#10666,#10667,#10668,#10669,
#10670,#10671,#10672,#10673,#10674,#10675,#10676,#10677,#10678,#10679,#10680,
#10681,#10682,#10683,#10684,#10685,#10686,#10687,#10688,#10689,#10690,#10691,
#10692,#10693,#10694,#10695,#10696,#10697,#10698,#10699,#10700,#10701,#10702,
#10703,#10704,#10705,#10706,#10707,#10708,#10709,#10710,#10711,#10712,#10713,
#10714,#10715,#10716,#10717,#10718,#10719,#10720,#10721,#10722,#10723,#10724,
#10725,#10726,#10727,#10728,#10729,#10730,#10731,#10732,#10733,#10734,#10735,
#10736,#10737,#10738,#10739,#10740,#10741,#10742,#10743,#10744,#10745,#10746,
#10747,#10748,#10749,#10750,#10751,#10752,#10753,#10754,#10755,#10756,#10757,
#10758,#10759,#10760,#10761,#10762,#10763,#10764,#10765,#10766,#10767,#10768,
#10769,#10770,#10771,#10772,#10773,#10774,#10775,#10776,#10777,#10778,#10779,
#10780,#10781,#10782,#10783,#10784,#10785,#10786,#10787,#10788,#10789,#10790,
#10791,#10792,#10793,#10794,#10795,#10796,#10797,#10798,#10799,#10800,#10801,
#10802,#10803,#10804,#10805,#10806,#10807,#10808,#10809,#10810,#10811,#10812,
#10813,#10814,#10815,#10816,#10817,#10818,#10819,#10820,#10821,#10822,#10823,
#10824,#10825,#10826,#10827,#10828));
#11712=AXIS2_PLACEMENT_3D('',#17191,#13900,#13901);
#11713=AXIS2_PLACEMENT_3D('',#17192,#13902,#13903);
#11714=AXIS2_PLACEMENT_3D('',#17195,#13904,#13905);
#11715=AXIS2_PLACEMENT_3D('',#17199,#13907,#13908);
#11716=AXIS2_PLACEMENT_3D('',#17201,#13910,#13911);
#11717=AXIS2_PLACEMENT_3D('',#17214,#13917,#13918);
#11718=AXIS2_PLACEMENT_3D('',#17218,#13920,#13921);
#11719=AXIS2_PLACEMENT_3D('',#17222,#13923,#13924);
#11720=AXIS2_PLACEMENT_3D('',#17226,#13926,#13927);
#11721=AXIS2_PLACEMENT_3D('',#17230,#13929,#13930);
#11722=AXIS2_PLACEMENT_3D('',#17234,#13932,#13933);
#11723=AXIS2_PLACEMENT_3D('',#17238,#13935,#13936);
#11724=AXIS2_PLACEMENT_3D('',#17242,#13938,#13939);
#11725=AXIS2_PLACEMENT_3D('',#17246,#13941,#13942);
#11726=AXIS2_PLACEMENT_3D('',#17250,#13944,#13945);
#11727=AXIS2_PLACEMENT_3D('',#17254,#13947,#13948);
#11728=AXIS2_PLACEMENT_3D('',#17272,#13957,#13958);
#11729=AXIS2_PLACEMENT_3D('',#17276,#13960,#13961);
#11730=AXIS2_PLACEMENT_3D('',#17280,#13963,#13964);
#11731=AXIS2_PLACEMENT_3D('',#17284,#13966,#13967);
#11732=AXIS2_PLACEMENT_3D('',#17288,#13969,#13970);
#11733=AXIS2_PLACEMENT_3D('',#17292,#13972,#13973);
#11734=AXIS2_PLACEMENT_3D('',#17296,#13975,#13976);
#11735=AXIS2_PLACEMENT_3D('',#17300,#13978,#13979);
#11736=AXIS2_PLACEMENT_3D('',#17304,#13981,#13982);
#11737=AXIS2_PLACEMENT_3D('',#17308,#13984,#13985);
#11738=AXIS2_PLACEMENT_3D('',#17312,#13987,#13988);
#11739=AXIS2_PLACEMENT_3D('',#17330,#13997,#13998);
#11740=AXIS2_PLACEMENT_3D('',#17334,#14000,#14001);
#11741=AXIS2_PLACEMENT_3D('',#17338,#14003,#14004);
#11742=AXIS2_PLACEMENT_3D('',#17342,#14006,#14007);
#11743=AXIS2_PLACEMENT_3D('',#17346,#14009,#14010);
#11744=AXIS2_PLACEMENT_3D('',#17350,#14012,#14013);
#11745=AXIS2_PLACEMENT_3D('',#17354,#14015,#14016);
#11746=AXIS2_PLACEMENT_3D('',#17358,#14018,#14019);
#11747=AXIS2_PLACEMENT_3D('',#17362,#14021,#14022);
#11748=AXIS2_PLACEMENT_3D('',#17366,#14024,#14025);
#11749=AXIS2_PLACEMENT_3D('',#17370,#14027,#14028);
#11750=AXIS2_PLACEMENT_3D('',#17388,#14037,#14038);
#11751=AXIS2_PLACEMENT_3D('',#17392,#14040,#14041);
#11752=AXIS2_PLACEMENT_3D('',#17396,#14043,#14044);
#11753=AXIS2_PLACEMENT_3D('',#17400,#14046,#14047);
#11754=AXIS2_PLACEMENT_3D('',#17404,#14049,#14050);
#11755=AXIS2_PLACEMENT_3D('',#17408,#14052,#14053);
#11756=AXIS2_PLACEMENT_3D('',#17412,#14055,#14056);
#11757=AXIS2_PLACEMENT_3D('',#17416,#14058,#14059);
#11758=AXIS2_PLACEMENT_3D('',#17420,#14061,#14062);
#11759=AXIS2_PLACEMENT_3D('',#17424,#14064,#14065);
#11760=AXIS2_PLACEMENT_3D('',#17428,#14067,#14068);
#11761=AXIS2_PLACEMENT_3D('',#17438,#14073,#14074);
#11762=AXIS2_PLACEMENT_3D('',#17442,#14076,#14077);
#11763=AXIS2_PLACEMENT_3D('',#17446,#14079,#14080);
#11764=AXIS2_PLACEMENT_3D('',#17449,#14082,#14083);
#11765=AXIS2_PLACEMENT_3D('',#17454,#14085,#14086);
#11766=AXIS2_PLACEMENT_3D('',#17458,#14088,#14089);
#11767=AXIS2_PLACEMENT_3D('',#17462,#14091,#14092);
#11768=AXIS2_PLACEMENT_3D('',#17466,#14094,#14095);
#11769=AXIS2_PLACEMENT_3D('',#17470,#14097,#14098);
#11770=AXIS2_PLACEMENT_3D('',#17474,#14100,#14101);
#11771=AXIS2_PLACEMENT_3D('',#17478,#14104,#14105);
#11772=AXIS2_PLACEMENT_3D('',#17483,#14107,#14108);
#11773=AXIS2_PLACEMENT_3D('',#17487,#14110,#14111);
#11774=AXIS2_PLACEMENT_3D('',#17491,#14113,#14114);
#11775=AXIS2_PLACEMENT_3D('',#17494,#14116,#14117);
#11776=AXIS2_PLACEMENT_3D('',#17499,#14119,#14120);
#11777=AXIS2_PLACEMENT_3D('',#17503,#14122,#14123);
#11778=AXIS2_PLACEMENT_3D('',#17507,#14125,#14126);
#11779=AXIS2_PLACEMENT_3D('',#17510,#14128,#14129);
#11780=AXIS2_PLACEMENT_3D('',#17515,#14131,#14132);
#11781=AXIS2_PLACEMENT_3D('',#17519,#14134,#14135);
#11782=AXIS2_PLACEMENT_3D('',#17523,#14137,#14138);
#11783=AXIS2_PLACEMENT_3D('',#17526,#14140,#14141);
#11784=AXIS2_PLACEMENT_3D('',#17527,#14142,#14143);
#11785=AXIS2_PLACEMENT_3D('',#17538,#14148,#14149);
#11786=AXIS2_PLACEMENT_3D('',#17542,#14151,#14152);
#11787=AXIS2_PLACEMENT_3D('',#17546,#14154,#14155);
#11788=AXIS2_PLACEMENT_3D('',#17550,#14157,#14158);
#11789=AXIS2_PLACEMENT_3D('',#17554,#14160,#14161);
#11790=AXIS2_PLACEMENT_3D('',#17558,#14163,#14164);
#11791=AXIS2_PLACEMENT_3D('',#17562,#14166,#14167);
#11792=AXIS2_PLACEMENT_3D('',#17566,#14169,#14170);
#11793=AXIS2_PLACEMENT_3D('',#17570,#14172,#14173);
#11794=AXIS2_PLACEMENT_3D('',#17574,#14175,#14176);
#11795=AXIS2_PLACEMENT_3D('',#17578,#14178,#14179);
#11796=AXIS2_PLACEMENT_3D('',#17596,#14188,#14189);
#11797=AXIS2_PLACEMENT_3D('',#17600,#14191,#14192);
#11798=AXIS2_PLACEMENT_3D('',#17604,#14194,#14195);
#11799=AXIS2_PLACEMENT_3D('',#17608,#14197,#14198);
#11800=AXIS2_PLACEMENT_3D('',#17612,#14200,#14201);
#11801=AXIS2_PLACEMENT_3D('',#17616,#14203,#14204);
#11802=AXIS2_PLACEMENT_3D('',#17620,#14206,#14207);
#11803=AXIS2_PLACEMENT_3D('',#17624,#14209,#14210);
#11804=AXIS2_PLACEMENT_3D('',#17628,#14212,#14213);
#11805=AXIS2_PLACEMENT_3D('',#17632,#14215,#14216);
#11806=AXIS2_PLACEMENT_3D('',#17636,#14218,#14219);
#11807=AXIS2_PLACEMENT_3D('',#17654,#14228,#14229);
#11808=AXIS2_PLACEMENT_3D('',#17658,#14231,#14232);
#11809=AXIS2_PLACEMENT_3D('',#17662,#14234,#14235);
#11810=AXIS2_PLACEMENT_3D('',#17666,#14237,#14238);
#11811=AXIS2_PLACEMENT_3D('',#17670,#14240,#14241);
#11812=AXIS2_PLACEMENT_3D('',#17674,#14243,#14244);
#11813=AXIS2_PLACEMENT_3D('',#17678,#14246,#14247);
#11814=AXIS2_PLACEMENT_3D('',#17682,#14249,#14250);
#11815=AXIS2_PLACEMENT_3D('',#17686,#14252,#14253);
#11816=AXIS2_PLACEMENT_3D('',#17690,#14255,#14256);
#11817=AXIS2_PLACEMENT_3D('',#17694,#14258,#14259);
#11818=AXIS2_PLACEMENT_3D('',#17712,#14268,#14269);
#11819=AXIS2_PLACEMENT_3D('',#17716,#14271,#14272);
#11820=AXIS2_PLACEMENT_3D('',#17720,#14274,#14275);
#11821=AXIS2_PLACEMENT_3D('',#17724,#14277,#14278);
#11822=AXIS2_PLACEMENT_3D('',#17728,#14280,#14281);
#11823=AXIS2_PLACEMENT_3D('',#17732,#14283,#14284);
#11824=AXIS2_PLACEMENT_3D('',#17736,#14286,#14287);
#11825=AXIS2_PLACEMENT_3D('',#17740,#14289,#14290);
#11826=AXIS2_PLACEMENT_3D('',#17744,#14292,#14293);
#11827=AXIS2_PLACEMENT_3D('',#17748,#14295,#14296);
#11828=AXIS2_PLACEMENT_3D('',#17752,#14298,#14299);
#11829=AXIS2_PLACEMENT_3D('',#17762,#14304,#14305);
#11830=AXIS2_PLACEMENT_3D('',#17766,#14307,#14308);
#11831=AXIS2_PLACEMENT_3D('',#17770,#14310,#14311);
#11832=AXIS2_PLACEMENT_3D('',#17774,#14313,#14314);
#11833=AXIS2_PLACEMENT_3D('',#17778,#14316,#14317);
#11834=AXIS2_PLACEMENT_3D('',#17782,#14319,#14320);
#11835=AXIS2_PLACEMENT_3D('',#17786,#14322,#14323);
#11836=AXIS2_PLACEMENT_3D('',#17790,#14325,#14326);
#11837=AXIS2_PLACEMENT_3D('',#17794,#14328,#14329);
#11838=AXIS2_PLACEMENT_3D('',#17798,#14331,#14332);
#11839=AXIS2_PLACEMENT_3D('',#17802,#14334,#14335);
#11840=AXIS2_PLACEMENT_3D('',#17806,#14337,#14338);
#11841=AXIS2_PLACEMENT_3D('',#17810,#14340,#14341);
#11842=AXIS2_PLACEMENT_3D('',#17814,#14343,#14344);
#11843=AXIS2_PLACEMENT_3D('',#17818,#14346,#14347);
#11844=AXIS2_PLACEMENT_3D('',#17822,#14349,#14350);
#11845=AXIS2_PLACEMENT_3D('',#17826,#14352,#14353);
#11846=AXIS2_PLACEMENT_3D('',#17830,#14355,#14356);
#11847=AXIS2_PLACEMENT_3D('',#17835,#14359,#14360);
#11848=AXIS2_PLACEMENT_3D('',#17839,#14362,#14363);
#11849=AXIS2_PLACEMENT_3D('',#17843,#14365,#14366);
#11850=AXIS2_PLACEMENT_3D('',#17847,#14368,#14369);
#11851=AXIS2_PLACEMENT_3D('',#17851,#14371,#14372);
#11852=AXIS2_PLACEMENT_3D('',#17853,#14374,#14375);
#11853=AXIS2_PLACEMENT_3D('',#17856,#14378,#14379);
#11854=AXIS2_PLACEMENT_3D('',#17858,#14381,#14382);
#11855=AXIS2_PLACEMENT_3D('',#17860,#14384,#14385);
#11856=AXIS2_PLACEMENT_3D('',#17862,#14387,#14388);
#11857=AXIS2_PLACEMENT_3D('',#17864,#14390,#14391);
#11858=AXIS2_PLACEMENT_3D('',#17866,#14393,#14394);
#11859=AXIS2_PLACEMENT_3D('',#17868,#14396,#14397);
#11860=AXIS2_PLACEMENT_3D('',#17870,#14399,#14400);
#11861=AXIS2_PLACEMENT_3D('',#17872,#14402,#14403);
#11862=AXIS2_PLACEMENT_3D('',#17874,#14405,#14406);
#11863=AXIS2_PLACEMENT_3D('',#17876,#14408,#14409);
#11864=AXIS2_PLACEMENT_3D('',#17878,#14411,#14412);
#11865=AXIS2_PLACEMENT_3D('',#17880,#14414,#14415);
#11866=AXIS2_PLACEMENT_3D('',#17882,#14417,#14418);
#11867=AXIS2_PLACEMENT_3D('',#17884,#14420,#14421);
#11868=AXIS2_PLACEMENT_3D('',#17886,#14423,#14424);
#11869=AXIS2_PLACEMENT_3D('',#17888,#14426,#14427);
#11870=AXIS2_PLACEMENT_3D('',#17890,#14429,#14430);
#11871=AXIS2_PLACEMENT_3D('',#17892,#14432,#14433);
#11872=AXIS2_PLACEMENT_3D('',#17894,#14435,#14436);
#11873=AXIS2_PLACEMENT_3D('',#17896,#14438,#14439);
#11874=AXIS2_PLACEMENT_3D('',#17898,#14441,#14442);
#11875=AXIS2_PLACEMENT_3D('',#17900,#14444,#14445);
#11876=AXIS2_PLACEMENT_3D('',#17902,#14447,#14448);
#11877=AXIS2_PLACEMENT_3D('',#17904,#14450,#14451);
#11878=AXIS2_PLACEMENT_3D('',#17906,#14453,#14454);
#11879=AXIS2_PLACEMENT_3D('',#17908,#14456,#14457);
#11880=AXIS2_PLACEMENT_3D('',#17910,#14459,#14460);
#11881=AXIS2_PLACEMENT_3D('',#17912,#14462,#14463);
#11882=AXIS2_PLACEMENT_3D('',#17914,#14465,#14466);
#11883=AXIS2_PLACEMENT_3D('',#17916,#14468,#14469);
#11884=AXIS2_PLACEMENT_3D('',#17918,#14471,#14472);
#11885=AXIS2_PLACEMENT_3D('',#17920,#14474,#14475);
#11886=AXIS2_PLACEMENT_3D('',#17922,#14477,#14478);
#11887=AXIS2_PLACEMENT_3D('',#17924,#14480,#14481);
#11888=AXIS2_PLACEMENT_3D('',#17926,#14483,#14484);
#11889=AXIS2_PLACEMENT_3D('',#17928,#14486,#14487);
#11890=AXIS2_PLACEMENT_3D('',#17930,#14489,#14490);
#11891=AXIS2_PLACEMENT_3D('',#17932,#14492,#14493);
#11892=AXIS2_PLACEMENT_3D('',#17934,#14495,#14496);
#11893=AXIS2_PLACEMENT_3D('',#17936,#14498,#14499);
#11894=AXIS2_PLACEMENT_3D('',#17938,#14501,#14502);
#11895=AXIS2_PLACEMENT_3D('',#17940,#14504,#14505);
#11896=AXIS2_PLACEMENT_3D('',#17942,#14507,#14508);
#11897=AXIS2_PLACEMENT_3D('',#17944,#14510,#14511);
#11898=AXIS2_PLACEMENT_3D('',#17946,#14513,#14514);
#11899=AXIS2_PLACEMENT_3D('',#17948,#14516,#14517);
#11900=AXIS2_PLACEMENT_3D('',#17950,#14519,#14520);
#11901=AXIS2_PLACEMENT_3D('',#17952,#14522,#14523);
#11902=AXIS2_PLACEMENT_3D('',#17954,#14525,#14526);
#11903=AXIS2_PLACEMENT_3D('',#17956,#14528,#14529);
#11904=AXIS2_PLACEMENT_3D('',#17958,#14531,#14532);
#11905=AXIS2_PLACEMENT_3D('',#17960,#14534,#14535);
#11906=AXIS2_PLACEMENT_3D('',#17962,#14537,#14538);
#11907=AXIS2_PLACEMENT_3D('',#17964,#14540,#14541);
#11908=AXIS2_PLACEMENT_3D('',#17966,#14543,#14544);
#11909=AXIS2_PLACEMENT_3D('',#17968,#14546,#14547);
#11910=AXIS2_PLACEMENT_3D('',#17970,#14549,#14550);
#11911=AXIS2_PLACEMENT_3D('',#17972,#14552,#14553);
#11912=AXIS2_PLACEMENT_3D('',#17974,#14555,#14556);
#11913=AXIS2_PLACEMENT_3D('',#17976,#14558,#14559);
#11914=AXIS2_PLACEMENT_3D('',#17978,#14561,#14562);
#11915=AXIS2_PLACEMENT_3D('',#17980,#14564,#14565);
#11916=AXIS2_PLACEMENT_3D('',#17982,#14567,#14568);
#11917=AXIS2_PLACEMENT_3D('',#17984,#14570,#14571);
#11918=AXIS2_PLACEMENT_3D('',#17986,#14573,#14574);
#11919=AXIS2_PLACEMENT_3D('',#17988,#14576,#14577);
#11920=AXIS2_PLACEMENT_3D('',#17990,#14579,#14580);
#11921=AXIS2_PLACEMENT_3D('',#17992,#14582,#14583);
#11922=AXIS2_PLACEMENT_3D('',#17994,#14585,#14586);
#11923=AXIS2_PLACEMENT_3D('',#17996,#14588,#14589);
#11924=AXIS2_PLACEMENT_3D('',#17998,#14591,#14592);
#11925=AXIS2_PLACEMENT_3D('',#18000,#14594,#14595);
#11926=AXIS2_PLACEMENT_3D('',#18002,#14597,#14598);
#11927=AXIS2_PLACEMENT_3D('',#18004,#14600,#14601);
#11928=AXIS2_PLACEMENT_3D('',#18006,#14603,#14604);
#11929=AXIS2_PLACEMENT_3D('',#18008,#14606,#14607);
#11930=AXIS2_PLACEMENT_3D('',#18010,#14609,#14610);
#11931=AXIS2_PLACEMENT_3D('',#18012,#14612,#14613);
#11932=AXIS2_PLACEMENT_3D('',#18014,#14615,#14616);
#11933=AXIS2_PLACEMENT_3D('',#18016,#14618,#14619);
#11934=AXIS2_PLACEMENT_3D('',#18018,#14621,#14622);
#11935=AXIS2_PLACEMENT_3D('',#18020,#14624,#14625);
#11936=AXIS2_PLACEMENT_3D('',#18022,#14627,#14628);
#11937=AXIS2_PLACEMENT_3D('',#18024,#14630,#14631);
#11938=AXIS2_PLACEMENT_3D('',#18026,#14633,#14634);
#11939=AXIS2_PLACEMENT_3D('',#18028,#14636,#14637);
#11940=AXIS2_PLACEMENT_3D('',#18030,#14639,#14640);
#11941=AXIS2_PLACEMENT_3D('',#18032,#14642,#14643);
#11942=AXIS2_PLACEMENT_3D('',#18034,#14645,#14646);
#11943=AXIS2_PLACEMENT_3D('',#18036,#14648,#14649);
#11944=AXIS2_PLACEMENT_3D('',#18038,#14651,#14652);
#11945=AXIS2_PLACEMENT_3D('',#18040,#14654,#14655);
#11946=AXIS2_PLACEMENT_3D('',#18042,#14657,#14658);
#11947=AXIS2_PLACEMENT_3D('',#18044,#14660,#14661);
#11948=AXIS2_PLACEMENT_3D('',#18046,#14663,#14664);
#11949=AXIS2_PLACEMENT_3D('',#18048,#14666,#14667);
#11950=AXIS2_PLACEMENT_3D('',#18050,#14669,#14670);
#11951=AXIS2_PLACEMENT_3D('',#18052,#14672,#14673);
#11952=AXIS2_PLACEMENT_3D('',#18054,#14675,#14676);
#11953=AXIS2_PLACEMENT_3D('',#18056,#14678,#14679);
#11954=AXIS2_PLACEMENT_3D('',#18058,#14681,#14682);
#11955=AXIS2_PLACEMENT_3D('',#18060,#14684,#14685);
#11956=AXIS2_PLACEMENT_3D('',#18062,#14687,#14688);
#11957=AXIS2_PLACEMENT_3D('',#18064,#14690,#14691);
#11958=AXIS2_PLACEMENT_3D('',#18066,#14693,#14694);
#11959=AXIS2_PLACEMENT_3D('',#18068,#14696,#14697);
#11960=AXIS2_PLACEMENT_3D('',#18070,#14699,#14700);
#11961=AXIS2_PLACEMENT_3D('',#18072,#14702,#14703);
#11962=AXIS2_PLACEMENT_3D('',#18074,#14705,#14706);
#11963=AXIS2_PLACEMENT_3D('',#18076,#14708,#14709);
#11964=AXIS2_PLACEMENT_3D('',#18078,#14711,#14712);
#11965=AXIS2_PLACEMENT_3D('',#18080,#14714,#14715);
#11966=AXIS2_PLACEMENT_3D('',#18082,#14717,#14718);
#11967=AXIS2_PLACEMENT_3D('',#18084,#14720,#14721);
#11968=AXIS2_PLACEMENT_3D('',#18085,#14722,#14723);
#11969=AXIS2_PLACEMENT_3D('',#18088,#14726,#14727);
#11970=AXIS2_PLACEMENT_3D('',#18090,#14729,#14730);
#11971=AXIS2_PLACEMENT_3D('',#18092,#14732,#14733);
#11972=AXIS2_PLACEMENT_3D('',#18094,#14735,#14736);
#11973=AXIS2_PLACEMENT_3D('',#18096,#14738,#14739);
#11974=AXIS2_PLACEMENT_3D('',#18098,#14741,#14742);
#11975=AXIS2_PLACEMENT_3D('',#18100,#14744,#14745);
#11976=AXIS2_PLACEMENT_3D('',#18101,#14746,#14747);
#11977=AXIS2_PLACEMENT_3D('',#18104,#14750,#14751);
#11978=AXIS2_PLACEMENT_3D('',#18106,#14753,#14754);
#11979=AXIS2_PLACEMENT_3D('',#18108,#14756,#14757);
#11980=AXIS2_PLACEMENT_3D('',#18109,#14758,#14759);
#11981=AXIS2_PLACEMENT_3D('',#18111,#14761,#14762);
#11982=AXIS2_PLACEMENT_3D('',#18113,#14764,#14765);
#11983=AXIS2_PLACEMENT_3D('',#18115,#14767,#14768);
#11984=AXIS2_PLACEMENT_3D('',#18117,#14770,#14771);
#11985=AXIS2_PLACEMENT_3D('',#18119,#14773,#14774);
#11986=AXIS2_PLACEMENT_3D('',#18121,#14776,#14777);
#11987=AXIS2_PLACEMENT_3D('',#18123,#14779,#14780);
#11988=AXIS2_PLACEMENT_3D('',#18125,#14782,#14783);
#11989=AXIS2_PLACEMENT_3D('',#18127,#14785,#14786);
#11990=AXIS2_PLACEMENT_3D('',#18129,#14788,#14789);
#11991=AXIS2_PLACEMENT_3D('',#18130,#14790,#14791);
#11992=AXIS2_PLACEMENT_3D('',#18133,#14794,#14795);
#11993=AXIS2_PLACEMENT_3D('',#18135,#14797,#14798);
#11994=AXIS2_PLACEMENT_3D('',#18137,#14800,#14801);
#11995=AXIS2_PLACEMENT_3D('',#18139,#14803,#14804);
#11996=AXIS2_PLACEMENT_3D('',#18141,#14806,#14807);
#11997=AXIS2_PLACEMENT_3D('',#18143,#14809,#14810);
#11998=AXIS2_PLACEMENT_3D('',#18145,#14812,#14813);
#11999=AXIS2_PLACEMENT_3D('',#18146,#14814,#14815);
#12000=AXIS2_PLACEMENT_3D('',#18149,#14818,#14819);
#12001=AXIS2_PLACEMENT_3D('',#18151,#14821,#14822);
#12002=AXIS2_PLACEMENT_3D('',#18153,#14824,#14825);
#12003=AXIS2_PLACEMENT_3D('',#18155,#14827,#14828);
#12004=AXIS2_PLACEMENT_3D('',#18157,#14830,#14831);
#12005=AXIS2_PLACEMENT_3D('',#18159,#14833,#14834);
#12006=AXIS2_PLACEMENT_3D('',#18161,#14836,#14837);
#12007=AXIS2_PLACEMENT_3D('',#18162,#14838,#14839);
#12008=AXIS2_PLACEMENT_3D('',#18165,#14842,#14843);
#12009=AXIS2_PLACEMENT_3D('',#18167,#14845,#14846);
#12010=AXIS2_PLACEMENT_3D('',#18169,#14848,#14849);
#12011=AXIS2_PLACEMENT_3D('',#18171,#14851,#14852);
#12012=AXIS2_PLACEMENT_3D('',#18173,#14854,#14855);
#12013=AXIS2_PLACEMENT_3D('',#18175,#14857,#14858);
#12014=AXIS2_PLACEMENT_3D('',#18177,#14860,#14861);
#13900=DIRECTION('axis',(0.,0.,1.));
#13901=DIRECTION('refdir',(1.,0.,0.));
#13902=DIRECTION('center_axis',(0.,0.,-1.));
#13903=DIRECTION('ref_axis',(-1.,0.,0.));
#13904=DIRECTION('center_axis',(0.,0.,1.));
#13905=DIRECTION('ref_axis',(1.,0.,0.));
#13906=DIRECTION('',(0.,0.,-1.));
#13907=DIRECTION('center_axis',(0.,0.,1.));
#13908=DIRECTION('ref_axis',(1.,0.,0.));
#13909=DIRECTION('',(0.,0.,-1.));
#13910=DIRECTION('center_axis',(0.,0.,1.));
#13911=DIRECTION('ref_axis',(1.,0.,0.));
#13912=DIRECTION('',(0.867884643612355,0.496765785236721,0.));
#13913=DIRECTION('',(0.867884643612355,-0.496765785236721,0.));
#13914=DIRECTION('',(1.,0.,0.));
#13915=DIRECTION('',(0.706716667923105,-0.707496679341793,0.));
#13916=DIRECTION('',(0.,-1.,0.));
#13917=DIRECTION('center_axis',(0.,0.,-1.));
#13918=DIRECTION('ref_axis',(1.,0.,0.));
#13919=DIRECTION('',(-1.,0.,0.));
#13920=DIRECTION('center_axis',(0.,0.,1.));
#13921=DIRECTION('ref_axis',(1.,0.,0.));
#13922=DIRECTION('',(1.54197609341422E-14,-1.,0.));
#13923=DIRECTION('center_axis',(0.,0.,1.));
#13924=DIRECTION('ref_axis',(1.,0.,0.));
#13925=DIRECTION('',(1.,0.,0.));
#13926=DIRECTION('center_axis',(0.,0.,-1.));
#13927=DIRECTION('ref_axis',(1.,0.,0.));
#13928=DIRECTION('',(0.,-1.,0.));
#13929=DIRECTION('center_axis',(0.,0.,1.));
#13930=DIRECTION('ref_axis',(1.,0.,0.));
#13931=DIRECTION('',(1.,1.68215601615235E-15,0.));
#13932=DIRECTION('center_axis',(0.,0.,1.));
#13933=DIRECTION('ref_axis',(1.,0.,0.));
#13934=DIRECTION('',(-1.68215592970338E-15,1.,0.));
#13935=DIRECTION('center_axis',(0.,0.,1.));
#13936=DIRECTION('ref_axis',(1.,0.,0.));
#13937=DIRECTION('',(-1.,1.38779120854827E-13,0.));
#13938=DIRECTION('center_axis',(0.,0.,-1.));
#13939=DIRECTION('ref_axis',(1.,0.,0.));
#13940=DIRECTION('',(0.,1.,0.));
#13941=DIRECTION('center_axis',(0.,0.,1.));
#13942=DIRECTION('ref_axis',(1.,0.,0.));
#13943=DIRECTION('',(-1.,-7.70988123297925E-15,0.));
#13944=DIRECTION('center_axis',(0.,0.,1.));
#13945=DIRECTION('ref_axis',(1.,0.,0.));
#13946=DIRECTION('',(0.,-1.,0.));
#13947=DIRECTION('center_axis',(0.,0.,-1.));
#13948=DIRECTION('ref_axis',(1.,0.,0.));
#13949=DIRECTION('',(-1.,2.72113516754055E-15,0.));
#13950=DIRECTION('',(-0.707106781186546,0.707106781186549,0.));
#13951=DIRECTION('',(0.,1.,0.));
#13952=DIRECTION('',(-0.499998732686741,0.866026135466853,0.));
#13953=DIRECTION('',(0.499998732686741,0.866026135466853,0.));
#13954=DIRECTION('',(0.,1.,0.));
#13955=DIRECTION('',(0.707106781186546,0.707106781186549,0.));
#13956=DIRECTION('',(1.,0.,0.));
#13957=DIRECTION('center_axis',(0.,0.,-1.));
#13958=DIRECTION('ref_axis',(1.,0.,0.));
#13959=DIRECTION('',(0.,-1.,0.));
#13960=DIRECTION('center_axis',(0.,0.,1.));
#13961=DIRECTION('ref_axis',(1.,0.,0.));
#13962=DIRECTION('',(1.,0.,0.));
#13963=DIRECTION('center_axis',(0.,0.,1.));
#13964=DIRECTION('ref_axis',(1.,0.,0.));
#13965=DIRECTION('',(0.,1.,0.));
#13966=DIRECTION('center_axis',(0.,0.,-1.));
#13967=DIRECTION('ref_axis',(1.,0.,0.));
#13968=DIRECTION('',(1.,6.93895604274136E-14,0.));
#13969=DIRECTION('center_axis',(0.,0.,1.));
#13970=DIRECTION('ref_axis',(1.,0.,0.));
#13971=DIRECTION('',(-1.68215592970338E-15,1.,0.));
#13972=DIRECTION('center_axis',(0.,0.,1.));
#13973=DIRECTION('ref_axis',(1.,0.,0.));
#13974=DIRECTION('',(-1.,0.,0.));
#13975=DIRECTION('center_axis',(0.,0.,1.));
#13976=DIRECTION('ref_axis',(1.,0.,0.));
#13977=DIRECTION('',(0.,-1.,0.));
#13978=DIRECTION('center_axis',(0.,0.,-1.));
#13979=DIRECTION('ref_axis',(1.,0.,0.));
#13980=DIRECTION('',(-1.,0.,0.));
#13981=DIRECTION('center_axis',(0.,0.,1.));
#13982=DIRECTION('ref_axis',(1.,0.,0.));
#13983=DIRECTION('',(0.,-1.,0.));
#13984=DIRECTION('center_axis',(0.,0.,1.));
#13985=DIRECTION('ref_axis',(1.,0.,0.));
#13986=DIRECTION('',(1.,-2.04085131219443E-15,0.));
#13987=DIRECTION('center_axis',(0.,0.,-1.));
#13988=DIRECTION('ref_axis',(1.,0.,0.));
#13989=DIRECTION('',(0.,-1.,0.));
#13990=DIRECTION('',(-0.706716667923105,-0.707496679341793,0.));
#13991=DIRECTION('',(-1.,0.,0.));
#13992=DIRECTION('',(-0.867884643612358,-0.496765785236715,0.));
#13993=DIRECTION('',(-0.867884643612358,0.496765785236715,0.));
#13994=DIRECTION('',(-1.,0.,0.));
#13995=DIRECTION('',(-0.706716667923105,0.707496679341793,0.));
#13996=DIRECTION('',(-5.4422705895004E-15,1.,0.));
#13997=DIRECTION('center_axis',(0.,0.,-1.));
#13998=DIRECTION('ref_axis',(1.,0.,0.));
#13999=DIRECTION('',(1.,0.,0.));
#14000=DIRECTION('center_axis',(0.,0.,1.));
#14001=DIRECTION('ref_axis',(1.,0.,0.));
#14002=DIRECTION('',(-1.54197609341422E-14,1.,0.));
#14003=DIRECTION('center_axis',(0.,0.,1.));
#14004=DIRECTION('ref_axis',(1.,0.,0.));
#14005=DIRECTION('',(-1.,0.,0.));
#14006=DIRECTION('center_axis',(0.,0.,-1.));
#14007=DIRECTION('ref_axis',(1.,0.,0.));
#14008=DIRECTION('',(0.,1.,0.));
#14009=DIRECTION('center_axis',(0.,0.,1.));
#14010=DIRECTION('ref_axis',(1.,0.,0.));
#14011=DIRECTION('',(-1.,-1.68215601615234E-15,0.));
#14012=DIRECTION('center_axis',(0.,0.,1.));
#14013=DIRECTION('ref_axis',(1.,0.,0.));
#14014=DIRECTION('',(1.68215592970338E-15,-1.,0.));
#14015=DIRECTION('center_axis',(0.,0.,1.));
#14016=DIRECTION('ref_axis',(1.,0.,0.));
#14017=DIRECTION('',(1.,-1.38779120854846E-13,0.));
#14018=DIRECTION('center_axis',(0.,0.,-1.));
#14019=DIRECTION('ref_axis',(1.,0.,0.));
#14020=DIRECTION('',(0.,-1.,0.));
#14021=DIRECTION('center_axis',(0.,0.,1.));
#14022=DIRECTION('ref_axis',(1.,0.,0.));
#14023=DIRECTION('',(1.,7.70988123297925E-15,0.));
#14024=DIRECTION('center_axis',(0.,0.,1.));
#14025=DIRECTION('ref_axis',(1.,0.,0.));
#14026=DIRECTION('',(-4.0817021727476E-15,1.,0.));
#14027=DIRECTION('center_axis',(0.,0.,-1.));
#14028=DIRECTION('ref_axis',(1.,0.,0.));
#14029=DIRECTION('',(1.,-2.72113516754055E-15,0.));
#14030=DIRECTION('',(0.707106781186547,-0.707106781186547,0.));
#14031=DIRECTION('',(0.,-1.,0.));
#14032=DIRECTION('',(0.499998732686731,-0.866026135466859,0.));
#14033=DIRECTION('',(-0.499998732686731,-0.866026135466859,0.));
#14034=DIRECTION('',(0.,-1.,0.));
#14035=DIRECTION('',(-0.707106781186547,-0.707106781186548,0.));
#14036=DIRECTION('',(-1.,0.,0.));
#14037=DIRECTION('center_axis',(0.,0.,-1.));
#14038=DIRECTION('ref_axis',(1.,0.,0.));
#14039=DIRECTION('',(0.,1.,0.));
#14040=DIRECTION('center_axis',(0.,0.,1.));
#14041=DIRECTION('ref_axis',(1.,0.,0.));
#14042=DIRECTION('',(-1.,-7.70988123297925E-15,0.));
#14043=DIRECTION('center_axis',(0.,0.,1.));
#14044=DIRECTION('ref_axis',(1.,0.,0.));
#14045=DIRECTION('',(0.,-1.,0.));
#14046=DIRECTION('center_axis',(0.,0.,-1.));
#14047=DIRECTION('ref_axis',(1.,0.,0.));
#14048=DIRECTION('',(-1.,-6.93895604274136E-14,0.));
#14049=DIRECTION('center_axis',(0.,0.,1.));
#14050=DIRECTION('ref_axis',(1.,0.,0.));
#14051=DIRECTION('',(1.68215592970338E-15,-1.,0.));
#14052=DIRECTION('center_axis',(0.,0.,1.));
#14053=DIRECTION('ref_axis',(1.,0.,0.));
#14054=DIRECTION('',(1.,0.,0.));
#14055=DIRECTION('center_axis',(0.,0.,1.));
#14056=DIRECTION('ref_axis',(1.,0.,0.));
#14057=DIRECTION('',(0.,1.,0.));
#14058=DIRECTION('center_axis',(0.,0.,-1.));
#14059=DIRECTION('ref_axis',(1.,0.,0.));
#14060=DIRECTION('',(1.,-3.46945490866966E-14,0.));
#14061=DIRECTION('center_axis',(0.,0.,1.));
#14062=DIRECTION('ref_axis',(1.,0.,0.));
#14063=DIRECTION('',(-1.54197609341422E-14,1.,0.));
#14064=DIRECTION('center_axis',(0.,0.,1.));
#14065=DIRECTION('ref_axis',(1.,0.,0.));
#14066=DIRECTION('',(-1.,1.0204256560972E-15,0.));
#14067=DIRECTION('center_axis',(0.,0.,-1.));
#14068=DIRECTION('ref_axis',(1.,0.,0.));
#14069=DIRECTION('',(0.,1.,0.));
#14070=DIRECTION('',(0.706716667923104,0.707496679341793,0.));
#14071=DIRECTION('',(1.,-2.09985316358847E-15,0.));
#14072=DIRECTION('',(-1.,0.,0.));
#14073=DIRECTION('center_axis',(0.,0.,1.));
#14074=DIRECTION('ref_axis',(1.,0.,0.));
#14075=DIRECTION('',(-6.30808317960405E-15,1.,0.));
#14076=DIRECTION('center_axis',(0.,0.,1.));
#14077=DIRECTION('ref_axis',(1.,0.,0.));
#14078=DIRECTION('',(1.,3.15404158980207E-15,0.));
#14079=DIRECTION('center_axis',(0.,0.,1.));
#14080=DIRECTION('ref_axis',(1.,0.,0.));
#14081=DIRECTION('',(0.,-1.,0.));
#14082=DIRECTION('center_axis',(0.,0.,1.));
#14083=DIRECTION('ref_axis',(1.,0.,0.));
#14084=DIRECTION('',(-0.778588686672397,0.627534586286487,0.));
#14085=DIRECTION('center_axis',(0.,0.,1.));
#14086=DIRECTION('ref_axis',(1.,0.,0.));
#14087=DIRECTION('',(-0.778588686672393,-0.627534586286492,0.));
#14088=DIRECTION('center_axis',(0.,0.,1.));
#14089=DIRECTION('ref_axis',(1.,0.,0.));
#14090=DIRECTION('',(0.61886791399197,0.785495070023503,0.));
#14091=DIRECTION('center_axis',(0.,0.,1.));
#14092=DIRECTION('ref_axis',(1.,0.,0.));
#14093=DIRECTION('',(-0.618867913991998,0.785495070023481,0.));
#14094=DIRECTION('center_axis',(0.,0.,1.));
#14095=DIRECTION('ref_axis',(1.,0.,0.));
#14096=DIRECTION('',(0.778588686672382,-0.627534586286505,0.));
#14097=DIRECTION('center_axis',(0.,0.,1.));
#14098=DIRECTION('ref_axis',(1.,0.,0.));
#14099=DIRECTION('',(0.778588686672372,0.627534586286517,0.));
#14100=DIRECTION('center_axis',(0.,0.,1.));
#14101=DIRECTION('ref_axis',(1.,0.,0.));
#14102=DIRECTION('',(-0.61886791399199,-0.785495070023487,0.));
#14103=DIRECTION('',(0.61886791399197,-0.785495070023503,0.));
#14104=DIRECTION('center_axis',(0.,0.,1.));
#14105=DIRECTION('ref_axis',(1.,0.,0.));
#14106=DIRECTION('',(1.,0.,0.));
#14107=DIRECTION('center_axis',(0.,0.,1.));
#14108=DIRECTION('ref_axis',(1.,0.,0.));
#14109=DIRECTION('',(6.30808317960409E-15,-1.,0.));
#14110=DIRECTION('center_axis',(0.,0.,1.));
#14111=DIRECTION('ref_axis',(1.,0.,0.));
#14112=DIRECTION('',(-1.,-3.15404158980205E-15,0.));
#14113=DIRECTION('center_axis',(0.,0.,1.));
#14114=DIRECTION('ref_axis',(1.,0.,0.));
#14115=DIRECTION('',(0.,1.,0.));
#14116=DIRECTION('center_axis',(0.,0.,1.));
#14117=DIRECTION('ref_axis',(1.,0.,0.));
#14118=DIRECTION('',(-6.30808317960404E-15,1.,0.));
#14119=DIRECTION('center_axis',(0.,0.,1.));
#14120=DIRECTION('ref_axis',(1.,0.,0.));
#14121=DIRECTION('',(1.,3.15404158980205E-15,0.));
#14122=DIRECTION('center_axis',(0.,0.,1.));
#14123=DIRECTION('ref_axis',(1.,0.,0.));
#14124=DIRECTION('',(0.,-1.,0.));
#14125=DIRECTION('center_axis',(0.,0.,1.));
#14126=DIRECTION('ref_axis',(1.,0.,0.));
#14127=DIRECTION('',(-1.,0.,0.));
#14128=DIRECTION('center_axis',(0.,0.,1.));
#14129=DIRECTION('ref_axis',(1.,0.,0.));
#14130=DIRECTION('',(-1.,0.,0.));
#14131=DIRECTION('center_axis',(0.,0.,1.));
#14132=DIRECTION('ref_axis',(1.,0.,0.));
#14133=DIRECTION('',(0.,1.,0.));
#14134=DIRECTION('center_axis',(0.,0.,1.));
#14135=DIRECTION('ref_axis',(1.,0.,0.));
#14136=DIRECTION('',(1.,0.,0.));
#14137=DIRECTION('center_axis',(0.,0.,1.));
#14138=DIRECTION('ref_axis',(1.,0.,0.));
#14139=DIRECTION('',(6.30808317960409E-15,-1.,0.));
#14140=DIRECTION('center_axis',(0.,0.,1.));
#14141=DIRECTION('ref_axis',(1.,0.,0.));
#14142=DIRECTION('center_axis',(0.,0.,1.));
#14143=DIRECTION('ref_axis',(1.,0.,0.));
#14144=DIRECTION('',(0.867884643612355,0.496765785236721,0.));
#14145=DIRECTION('',(1.,-2.09985316358847E-15,0.));
#14146=DIRECTION('',(0.706716667923104,0.707496679341793,0.));
#14147=DIRECTION('',(0.,1.,0.));
#14148=DIRECTION('center_axis',(0.,0.,-1.));
#14149=DIRECTION('ref_axis',(1.,0.,0.));
#14150=DIRECTION('',(-1.,1.0204256560972E-15,0.));
#14151=DIRECTION('center_axis',(0.,0.,1.));
#14152=DIRECTION('ref_axis',(1.,0.,0.));
#14153=DIRECTION('',(-1.54197609341422E-14,1.,0.));
#14154=DIRECTION('center_axis',(0.,0.,1.));
#14155=DIRECTION('ref_axis',(1.,0.,0.));
#14156=DIRECTION('',(1.,-3.46945490866966E-14,0.));
#14157=DIRECTION('center_axis',(0.,0.,-1.));
#14158=DIRECTION('ref_axis',(1.,0.,0.));
#14159=DIRECTION('',(0.,1.,0.));
#14160=DIRECTION('center_axis',(0.,0.,1.));
#14161=DIRECTION('ref_axis',(1.,0.,0.));
#14162=DIRECTION('',(1.,0.,0.));
#14163=DIRECTION('center_axis',(0.,0.,1.));
#14164=DIRECTION('ref_axis',(1.,0.,0.));
#14165=DIRECTION('',(1.68215592970338E-15,-1.,0.));
#14166=DIRECTION('center_axis',(0.,0.,1.));
#14167=DIRECTION('ref_axis',(1.,0.,0.));
#14168=DIRECTION('',(-1.,-6.93895604274136E-14,0.));
#14169=DIRECTION('center_axis',(0.,0.,-1.));
#14170=DIRECTION('ref_axis',(1.,0.,0.));
#14171=DIRECTION('',(0.,-1.,0.));
#14172=DIRECTION('center_axis',(0.,0.,1.));
#14173=DIRECTION('ref_axis',(1.,0.,0.));
#14174=DIRECTION('',(-1.,-7.70988123297925E-15,0.));
#14175=DIRECTION('center_axis',(0.,0.,1.));
#14176=DIRECTION('ref_axis',(1.,0.,0.));
#14177=DIRECTION('',(0.,1.,0.));
#14178=DIRECTION('center_axis',(0.,0.,-1.));
#14179=DIRECTION('ref_axis',(1.,0.,0.));
#14180=DIRECTION('',(-1.,0.,0.));
#14181=DIRECTION('',(-0.707106781186547,-0.707106781186548,0.));
#14182=DIRECTION('',(0.,-1.,0.));
#14183=DIRECTION('',(-0.499998732686731,-0.866026135466859,0.));
#14184=DIRECTION('',(0.499998732686731,-0.866026135466859,0.));
#14185=DIRECTION('',(0.,-1.,0.));
#14186=DIRECTION('',(0.707106781186547,-0.707106781186547,0.));
#14187=DIRECTION('',(1.,-2.72113516754055E-15,0.));
#14188=DIRECTION('center_axis',(0.,0.,-1.));
#14189=DIRECTION('ref_axis',(1.,0.,0.));
#14190=DIRECTION('',(-4.0817021727476E-15,1.,0.));
#14191=DIRECTION('center_axis',(0.,0.,1.));
#14192=DIRECTION('ref_axis',(1.,0.,0.));
#14193=DIRECTION('',(1.,7.70988123297925E-15,0.));
#14194=DIRECTION('center_axis',(0.,0.,1.));
#14195=DIRECTION('ref_axis',(1.,0.,0.));
#14196=DIRECTION('',(0.,-1.,0.));
#14197=DIRECTION('center_axis',(0.,0.,-1.));
#14198=DIRECTION('ref_axis',(1.,0.,0.));
#14199=DIRECTION('',(1.,-1.38779120854846E-13,0.));
#14200=DIRECTION('center_axis',(0.,0.,1.));
#14201=DIRECTION('ref_axis',(1.,0.,0.));
#14202=DIRECTION('',(1.68215592970338E-15,-1.,0.));
#14203=DIRECTION('center_axis',(0.,0.,1.));
#14204=DIRECTION('ref_axis',(1.,0.,0.));
#14205=DIRECTION('',(-1.,-1.68215601615234E-15,0.));
#14206=DIRECTION('center_axis',(0.,0.,1.));
#14207=DIRECTION('ref_axis',(1.,0.,0.));
#14208=DIRECTION('',(0.,1.,0.));
#14209=DIRECTION('center_axis',(0.,0.,-1.));
#14210=DIRECTION('ref_axis',(1.,0.,0.));
#14211=DIRECTION('',(-1.,0.,0.));
#14212=DIRECTION('center_axis',(0.,0.,1.));
#14213=DIRECTION('ref_axis',(1.,0.,0.));
#14214=DIRECTION('',(-1.54197609341422E-14,1.,0.));
#14215=DIRECTION('center_axis',(0.,0.,1.));
#14216=DIRECTION('ref_axis',(1.,0.,0.));
#14217=DIRECTION('',(1.,0.,0.));
#14218=DIRECTION('center_axis',(0.,0.,-1.));
#14219=DIRECTION('ref_axis',(1.,0.,0.));
#14220=DIRECTION('',(-5.4422705895004E-15,1.,0.));
#14221=DIRECTION('',(-0.706716667923105,0.707496679341793,0.));
#14222=DIRECTION('',(-1.,0.,0.));
#14223=DIRECTION('',(-0.867884643612358,0.496765785236715,0.));
#14224=DIRECTION('',(-0.867884643612358,-0.496765785236715,0.));
#14225=DIRECTION('',(-1.,0.,0.));
#14226=DIRECTION('',(-0.706716667923105,-0.707496679341793,0.));
#14227=DIRECTION('',(0.,-1.,0.));
#14228=DIRECTION('center_axis',(0.,0.,-1.));
#14229=DIRECTION('ref_axis',(1.,0.,0.));
#14230=DIRECTION('',(1.,-2.04085131219443E-15,0.));
#14231=DIRECTION('center_axis',(0.,0.,1.));
#14232=DIRECTION('ref_axis',(1.,0.,0.));
#14233=DIRECTION('',(0.,-1.,0.));
#14234=DIRECTION('center_axis',(0.,0.,1.));
#14235=DIRECTION('ref_axis',(1.,0.,0.));
#14236=DIRECTION('',(-1.,0.,0.));
#14237=DIRECTION('center_axis',(0.,0.,-1.));
#14238=DIRECTION('ref_axis',(1.,0.,0.));
#14239=DIRECTION('',(0.,-1.,0.));
#14240=DIRECTION('center_axis',(0.,0.,1.));
#14241=DIRECTION('ref_axis',(1.,0.,0.));
#14242=DIRECTION('',(-1.,0.,0.));
#14243=DIRECTION('center_axis',(0.,0.,1.));
#14244=DIRECTION('ref_axis',(1.,0.,0.));
#14245=DIRECTION('',(-1.68215592970338E-15,1.,0.));
#14246=DIRECTION('center_axis',(0.,0.,1.));
#14247=DIRECTION('ref_axis',(1.,0.,0.));
#14248=DIRECTION('',(1.,6.93895604274136E-14,0.));
#14249=DIRECTION('center_axis',(0.,0.,-1.));
#14250=DIRECTION('ref_axis',(1.,0.,0.));
#14251=DIRECTION('',(0.,1.,0.));
#14252=DIRECTION('center_axis',(0.,0.,1.));
#14253=DIRECTION('ref_axis',(1.,0.,0.));
#14254=DIRECTION('',(1.,0.,0.));
#14255=DIRECTION('center_axis',(0.,0.,1.));
#14256=DIRECTION('ref_axis',(1.,0.,0.));
#14257=DIRECTION('',(0.,-1.,0.));
#14258=DIRECTION('center_axis',(0.,0.,-1.));
#14259=DIRECTION('ref_axis',(1.,0.,0.));
#14260=DIRECTION('',(1.,0.,0.));
#14261=DIRECTION('',(0.707106781186546,0.707106781186549,0.));
#14262=DIRECTION('',(0.,1.,0.));
#14263=DIRECTION('',(0.499998732686741,0.866026135466853,0.));
#14264=DIRECTION('',(-0.499998732686741,0.866026135466853,0.));
#14265=DIRECTION('',(0.,1.,0.));
#14266=DIRECTION('',(-0.707106781186546,0.707106781186549,0.));
#14267=DIRECTION('',(-1.,2.72113516754055E-15,0.));
#14268=DIRECTION('center_axis',(0.,0.,-1.));
#14269=DIRECTION('ref_axis',(1.,0.,0.));
#14270=DIRECTION('',(0.,-1.,0.));
#14271=DIRECTION('center_axis',(0.,0.,1.));
#14272=DIRECTION('ref_axis',(1.,0.,0.));
#14273=DIRECTION('',(-1.,-7.70988123297925E-15,0.));
#14274=DIRECTION('center_axis',(0.,0.,1.));
#14275=DIRECTION('ref_axis',(1.,0.,0.));
#14276=DIRECTION('',(0.,1.,0.));
#14277=DIRECTION('center_axis',(0.,0.,-1.));
#14278=DIRECTION('ref_axis',(1.,0.,0.));
#14279=DIRECTION('',(-1.,1.38779120854827E-13,0.));
#14280=DIRECTION('center_axis',(0.,0.,1.));
#14281=DIRECTION('ref_axis',(1.,0.,0.));
#14282=DIRECTION('',(-1.68215592970338E-15,1.,0.));
#14283=DIRECTION('center_axis',(0.,0.,1.));
#14284=DIRECTION('ref_axis',(1.,0.,0.));
#14285=DIRECTION('',(1.,1.68215601615235E-15,0.));
#14286=DIRECTION('center_axis',(0.,0.,1.));
#14287=DIRECTION('ref_axis',(1.,0.,0.));
#14288=DIRECTION('',(0.,-1.,0.));
#14289=DIRECTION('center_axis',(0.,0.,-1.));
#14290=DIRECTION('ref_axis',(1.,0.,0.));
#14291=DIRECTION('',(1.,0.,0.));
#14292=DIRECTION('center_axis',(0.,0.,1.));
#14293=DIRECTION('ref_axis',(1.,0.,0.));
#14294=DIRECTION('',(1.54197609341422E-14,-1.,0.));
#14295=DIRECTION('center_axis',(0.,0.,1.));
#14296=DIRECTION('ref_axis',(1.,0.,0.));
#14297=DIRECTION('',(-1.,0.,0.));
#14298=DIRECTION('center_axis',(0.,0.,-1.));
#14299=DIRECTION('ref_axis',(1.,0.,0.));
#14300=DIRECTION('',(0.,-1.,0.));
#14301=DIRECTION('',(0.706716667923105,-0.707496679341793,0.));
#14302=DIRECTION('',(1.,0.,0.));
#14303=DIRECTION('',(0.867884643612355,-0.496765785236721,0.));
#14304=DIRECTION('center_axis',(0.,0.,1.));
#14305=DIRECTION('ref_axis',(1.,0.,0.));
#14306=DIRECTION('',(-1.,0.,0.));
#14307=DIRECTION('center_axis',(0.,0.,1.));
#14308=DIRECTION('ref_axis',(1.,0.,0.));
#14309=DIRECTION('',(0.,-1.,0.));
#14310=DIRECTION('center_axis',(0.,0.,1.));
#14311=DIRECTION('ref_axis',(1.,0.,0.));
#14312=DIRECTION('',(1.,3.15404158980207E-15,0.));
#14313=DIRECTION('center_axis',(0.,0.,1.));
#14314=DIRECTION('ref_axis',(1.,0.,0.));
#14315=DIRECTION('',(-6.30808317960405E-15,1.,0.));
#14316=DIRECTION('center_axis',(0.,0.,1.));
#14317=DIRECTION('ref_axis',(1.,0.,0.));
#14318=DIRECTION('',(1.,0.,0.));
#14319=DIRECTION('center_axis',(0.,0.,1.));
#14320=DIRECTION('ref_axis',(1.,0.,0.));
#14321=DIRECTION('',(0.,1.,0.));
#14322=DIRECTION('center_axis',(0.,0.,1.));
#14323=DIRECTION('ref_axis',(1.,0.,0.));
#14324=DIRECTION('',(-1.,-3.15404158980205E-15,0.));
#14325=DIRECTION('center_axis',(0.,0.,1.));
#14326=DIRECTION('ref_axis',(1.,0.,0.));
#14327=DIRECTION('',(6.30808317960409E-15,-1.,0.));
#14328=DIRECTION('center_axis',(0.,0.,1.));
#14329=DIRECTION('ref_axis',(1.,0.,0.));
#14330=DIRECTION('',(-1.,0.,0.));
#14331=DIRECTION('center_axis',(0.,0.,1.));
#14332=DIRECTION('ref_axis',(1.,0.,0.));
#14333=DIRECTION('',(6.30808317960409E-15,-1.,0.));
#14334=DIRECTION('center_axis',(0.,0.,1.));
#14335=DIRECTION('ref_axis',(1.,0.,0.));
#14336=DIRECTION('',(1.,0.,0.));
#14337=DIRECTION('center_axis',(0.,0.,1.));
#14338=DIRECTION('ref_axis',(1.,0.,0.));
#14339=DIRECTION('',(0.,1.,0.));
#14340=DIRECTION('center_axis',(0.,0.,1.));
#14341=DIRECTION('ref_axis',(1.,0.,0.));
#14342=DIRECTION('',(-6.30808317960404E-15,1.,0.));
#14343=DIRECTION('center_axis',(0.,0.,1.));
#14344=DIRECTION('ref_axis',(1.,0.,0.));
#14345=DIRECTION('',(-1.,0.,0.));
#14346=DIRECTION('center_axis',(0.,0.,1.));
#14347=DIRECTION('ref_axis',(1.,0.,0.));
#14348=DIRECTION('',(0.,-1.,0.));
#14349=DIRECTION('center_axis',(0.,0.,1.));
#14350=DIRECTION('ref_axis',(1.,0.,0.));
#14351=DIRECTION('',(1.,3.15404158980205E-15,0.));
#14352=DIRECTION('center_axis',(0.,0.,1.));
#14353=DIRECTION('ref_axis',(1.,0.,0.));
#14354=DIRECTION('',(-0.778588686672397,0.627534586286487,0.));
#14355=DIRECTION('center_axis',(0.,0.,1.));
#14356=DIRECTION('ref_axis',(1.,0.,0.));
#14357=DIRECTION('',(0.61886791399197,-0.785495070023503,0.));
#14358=DIRECTION('',(-0.61886791399199,-0.785495070023487,0.));
#14359=DIRECTION('center_axis',(0.,0.,1.));
#14360=DIRECTION('ref_axis',(1.,0.,0.));
#14361=DIRECTION('',(0.778588686672372,0.627534586286517,0.));
#14362=DIRECTION('center_axis',(0.,0.,1.));
#14363=DIRECTION('ref_axis',(1.,0.,0.));
#14364=DIRECTION('',(0.778588686672382,-0.627534586286505,0.));
#14365=DIRECTION('center_axis',(0.,0.,1.));
#14366=DIRECTION('ref_axis',(1.,0.,0.));
#14367=DIRECTION('',(-0.618867913991998,0.785495070023481,0.));
#14368=DIRECTION('center_axis',(0.,0.,1.));
#14369=DIRECTION('ref_axis',(1.,0.,0.));
#14370=DIRECTION('',(0.61886791399197,0.785495070023503,0.));
#14371=DIRECTION('center_axis',(0.,0.,1.));
#14372=DIRECTION('ref_axis',(1.,0.,0.));
#14373=DIRECTION('',(-0.778588686672393,-0.627534586286492,0.));
#14374=DIRECTION('center_axis',(-0.496765785236721,0.867884643612355,0.));
#14375=DIRECTION('ref_axis',(-0.867884643612355,-0.496765785236721,0.));
#14376=DIRECTION('',(0.,0.,-1.));
#14377=DIRECTION('',(0.,0.,-1.));
#14378=DIRECTION('center_axis',(0.496765785236721,0.867884643612355,0.));
#14379=DIRECTION('ref_axis',(-0.867884643612355,0.496765785236721,0.));
#14380=DIRECTION('',(0.,0.,-1.));
#14381=DIRECTION('center_axis',(0.,1.,0.));
#14382=DIRECTION('ref_axis',(0.,0.,1.));
#14383=DIRECTION('',(0.,0.,-1.));
#14384=DIRECTION('center_axis',(0.707496679341793,0.706716667923105,0.));
#14385=DIRECTION('ref_axis',(-0.706716667923105,0.707496679341793,0.));
#14386=DIRECTION('',(0.,0.,-1.));
#14387=DIRECTION('center_axis',(1.,0.,0.));
#14388=DIRECTION('ref_axis',(0.,0.,-1.));
#14389=DIRECTION('',(0.,0.,-1.));
#14390=DIRECTION('center_axis',(0.,0.,-1.));
#14391=DIRECTION('ref_axis',(-1.,0.,0.));
#14392=DIRECTION('',(0.,0.,-1.));
#14393=DIRECTION('center_axis',(0.,-1.,0.));
#14394=DIRECTION('ref_axis',(0.,0.,-1.));
#14395=DIRECTION('',(0.,0.,-1.));
#14396=DIRECTION('center_axis',(0.,0.,-1.));
#14397=DIRECTION('ref_axis',(-1.,0.,0.));
#14398=DIRECTION('',(0.,0.,-1.));
#14399=DIRECTION('center_axis',(1.,1.54197609341421E-14,0.));
#14400=DIRECTION('ref_axis',(-1.54197609341421E-14,1.,0.));
#14401=DIRECTION('',(0.,0.,-1.));
#14402=DIRECTION('center_axis',(0.,0.,-1.));
#14403=DIRECTION('ref_axis',(-1.,0.,0.));
#14404=DIRECTION('',(0.,0.,-1.));
#14405=DIRECTION('center_axis',(0.,1.,0.));
#14406=DIRECTION('ref_axis',(0.,0.,1.));
#14407=DIRECTION('',(0.,0.,-1.));
#14408=DIRECTION('center_axis',(0.,0.,-1.));
#14409=DIRECTION('ref_axis',(-1.,0.,0.));
#14410=DIRECTION('',(0.,0.,-1.));
#14411=DIRECTION('center_axis',(1.,0.,0.));
#14412=DIRECTION('ref_axis',(0.,0.,-1.));
#14413=DIRECTION('',(0.,0.,-1.));
#14414=DIRECTION('center_axis',(0.,0.,-1.));
#14415=DIRECTION('ref_axis',(-1.,0.,0.));
#14416=DIRECTION('',(0.,0.,-1.));
#14417=DIRECTION('center_axis',(-1.68215601615235E-15,1.,0.));
#14418=DIRECTION('ref_axis',(-1.,-1.68215601615235E-15,0.));
#14419=DIRECTION('',(0.,0.,-1.));
#14420=DIRECTION('center_axis',(0.,0.,-1.));
#14421=DIRECTION('ref_axis',(-1.,0.,0.));
#14422=DIRECTION('',(0.,0.,-1.));
#14423=DIRECTION('center_axis',(-1.,-1.68215592970338E-15,0.));
#14424=DIRECTION('ref_axis',(1.68215592970338E-15,-1.,0.));
#14425=DIRECTION('',(0.,0.,-1.));
#14426=DIRECTION('center_axis',(0.,0.,-1.));
#14427=DIRECTION('ref_axis',(-1.,0.,0.));
#14428=DIRECTION('',(0.,0.,-1.));
#14429=DIRECTION('center_axis',(-1.38779120854827E-13,-1.,0.));
#14430=DIRECTION('ref_axis',(1.,-1.38779120854827E-13,0.));
#14431=DIRECTION('',(0.,0.,-1.));
#14432=DIRECTION('center_axis',(0.,0.,-1.));
#14433=DIRECTION('ref_axis',(-1.,0.,0.));
#14434=DIRECTION('',(0.,0.,-1.));
#14435=DIRECTION('center_axis',(-1.,0.,0.));
#14436=DIRECTION('ref_axis',(0.,0.,1.));
#14437=DIRECTION('',(0.,0.,-1.));
#14438=DIRECTION('center_axis',(0.,0.,-1.));
#14439=DIRECTION('ref_axis',(-1.,0.,0.));
#14440=DIRECTION('',(0.,0.,-1.));
#14441=DIRECTION('center_axis',(7.70988123297925E-15,-1.,0.));
#14442=DIRECTION('ref_axis',(1.,7.70988123297925E-15,0.));
#14443=DIRECTION('',(0.,0.,-1.));
#14444=DIRECTION('center_axis',(0.,0.,-1.));
#14445=DIRECTION('ref_axis',(-1.,0.,0.));
#14446=DIRECTION('',(0.,0.,-1.));
#14447=DIRECTION('center_axis',(1.,0.,0.));
#14448=DIRECTION('ref_axis',(0.,0.,-1.));
#14449=DIRECTION('',(0.,0.,-1.));
#14450=DIRECTION('center_axis',(0.,0.,-1.));
#14451=DIRECTION('ref_axis',(-1.,0.,0.));
#14452=DIRECTION('',(0.,0.,-1.));
#14453=DIRECTION('center_axis',(-2.72113516754055E-15,-1.,0.));
#14454=DIRECTION('ref_axis',(1.,-2.72113516754055E-15,0.));
#14455=DIRECTION('',(0.,0.,-1.));
#14456=DIRECTION('center_axis',(-0.707106781186549,-0.707106781186546,0.));
#14457=DIRECTION('ref_axis',(0.707106781186546,-0.707106781186549,0.));
#14458=DIRECTION('',(0.,0.,-1.));
#14459=DIRECTION('center_axis',(-1.,0.,0.));
#14460=DIRECTION('ref_axis',(0.,0.,1.));
#14461=DIRECTION('',(0.,0.,-1.));
#14462=DIRECTION('center_axis',(-0.866026135466853,-0.499998732686741,0.));
#14463=DIRECTION('ref_axis',(0.499998732686741,-0.866026135466854,0.));
#14464=DIRECTION('',(0.,0.,-1.));
#14465=DIRECTION('center_axis',(-0.866026135466853,0.499998732686741,0.));
#14466=DIRECTION('ref_axis',(-0.499998732686741,-0.866026135466854,0.));
#14467=DIRECTION('',(0.,0.,-1.));
#14468=DIRECTION('center_axis',(-1.,0.,0.));
#14469=DIRECTION('ref_axis',(0.,0.,1.));
#14470=DIRECTION('',(0.,0.,-1.));
#14471=DIRECTION('center_axis',(-0.707106781186549,0.707106781186546,0.));
#14472=DIRECTION('ref_axis',(-0.707106781186546,-0.707106781186549,0.));
#14473=DIRECTION('',(0.,0.,-1.));
#14474=DIRECTION('center_axis',(0.,1.,0.));
#14475=DIRECTION('ref_axis',(0.,0.,1.));
#14476=DIRECTION('',(0.,0.,-1.));
#14477=DIRECTION('center_axis',(0.,0.,-1.));
#14478=DIRECTION('ref_axis',(-1.,0.,0.));
#14479=DIRECTION('',(0.,0.,-1.));
#14480=DIRECTION('center_axis',(1.,0.,0.));
#14481=DIRECTION('ref_axis',(0.,0.,-1.));
#14482=DIRECTION('',(0.,0.,-1.));
#14483=DIRECTION('center_axis',(0.,0.,-1.));
#14484=DIRECTION('ref_axis',(-1.,0.,0.));
#14485=DIRECTION('',(0.,0.,-1.));
#14486=DIRECTION('center_axis',(0.,1.,0.));
#14487=DIRECTION('ref_axis',(0.,0.,1.));
#14488=DIRECTION('',(0.,0.,-1.));
#14489=DIRECTION('center_axis',(0.,0.,-1.));
#14490=DIRECTION('ref_axis',(-1.,0.,0.));
#14491=DIRECTION('',(0.,0.,-1.));
#14492=DIRECTION('center_axis',(-1.,0.,0.));
#14493=DIRECTION('ref_axis',(0.,0.,1.));
#14494=DIRECTION('',(0.,0.,-1.));
#14495=DIRECTION('center_axis',(0.,0.,-1.));
#14496=DIRECTION('ref_axis',(-1.,0.,0.));
#14497=DIRECTION('',(0.,0.,-1.));
#14498=DIRECTION('center_axis',(-6.93895604274136E-14,1.,0.));
#14499=DIRECTION('ref_axis',(-1.,-6.93895604274136E-14,0.));
#14500=DIRECTION('',(0.,0.,-1.));
#14501=DIRECTION('center_axis',(0.,0.,-1.));
#14502=DIRECTION('ref_axis',(-1.,0.,0.));
#14503=DIRECTION('',(0.,0.,-1.));
#14504=DIRECTION('center_axis',(-1.,-1.68215592970338E-15,0.));
#14505=DIRECTION('ref_axis',(1.68215592970338E-15,-1.,0.));
#14506=DIRECTION('',(0.,0.,-1.));
#14507=DIRECTION('center_axis',(0.,0.,-1.));
#14508=DIRECTION('ref_axis',(-1.,0.,0.));
#14509=DIRECTION('',(0.,0.,-1.));
#14510=DIRECTION('center_axis',(0.,-1.,0.));
#14511=DIRECTION('ref_axis',(0.,0.,-1.));
#14512=DIRECTION('',(0.,0.,-1.));
#14513=DIRECTION('center_axis',(0.,0.,-1.));
#14514=DIRECTION('ref_axis',(-1.,0.,0.));
#14515=DIRECTION('',(0.,0.,-1.));
#14516=DIRECTION('center_axis',(1.,0.,0.));
#14517=DIRECTION('ref_axis',(0.,0.,-1.));
#14518=DIRECTION('',(0.,0.,-1.));
#14519=DIRECTION('center_axis',(0.,0.,-1.));
#14520=DIRECTION('ref_axis',(-1.,0.,0.));
#14521=DIRECTION('',(0.,0.,-1.));
#14522=DIRECTION('center_axis',(0.,-1.,0.));
#14523=DIRECTION('ref_axis',(0.,0.,-1.));
#14524=DIRECTION('',(0.,0.,-1.));
#14525=DIRECTION('center_axis',(0.,0.,-1.));
#14526=DIRECTION('ref_axis',(-1.,0.,0.));
#14527=DIRECTION('',(0.,0.,-1.));
#14528=DIRECTION('center_axis',(1.,0.,0.));
#14529=DIRECTION('ref_axis',(0.,0.,-1.));
#14530=DIRECTION('',(0.,0.,-1.));
#14531=DIRECTION('center_axis',(0.,0.,-1.));
#14532=DIRECTION('ref_axis',(-1.,0.,0.));
#14533=DIRECTION('',(0.,0.,-1.));
#14534=DIRECTION('center_axis',(2.04085131219443E-15,1.,0.));
#14535=DIRECTION('ref_axis',(-1.,2.04085131219443E-15,0.));
#14536=DIRECTION('',(0.,0.,-1.));
#14537=DIRECTION('center_axis',(0.,0.,-1.));
#14538=DIRECTION('ref_axis',(-1.,0.,0.));
#14539=DIRECTION('',(0.,0.,-1.));
#14540=DIRECTION('center_axis',(1.,0.,0.));
#14541=DIRECTION('ref_axis',(0.,0.,-1.));
#14542=DIRECTION('',(0.,0.,-1.));
#14543=DIRECTION('center_axis',(0.707496679341793,-0.706716667923105,0.));
#14544=DIRECTION('ref_axis',(0.706716667923105,0.707496679341793,0.));
#14545=DIRECTION('',(0.,0.,-1.));
#14546=DIRECTION('center_axis',(0.,-1.,0.));
#14547=DIRECTION('ref_axis',(0.,0.,-1.));
#14548=DIRECTION('',(0.,0.,-1.));
#14549=DIRECTION('center_axis',(0.496765785236716,-0.867884643612358,0.));
#14550=DIRECTION('ref_axis',(0.867884643612358,0.496765785236716,0.));
#14551=DIRECTION('',(0.,0.,-1.));
#14552=DIRECTION('center_axis',(-0.496765785236716,-0.867884643612358,0.));
#14553=DIRECTION('ref_axis',(0.867884643612358,-0.496765785236716,0.));
#14554=DIRECTION('',(0.,0.,-1.));
#14555=DIRECTION('center_axis',(0.,-1.,0.));
#14556=DIRECTION('ref_axis',(0.,0.,-1.));
#14557=DIRECTION('',(0.,0.,-1.));
#14558=DIRECTION('center_axis',(-0.707496679341793,-0.706716667923105,0.));
#14559=DIRECTION('ref_axis',(0.706716667923105,-0.707496679341793,0.));
#14560=DIRECTION('',(0.,0.,-1.));
#14561=DIRECTION('center_axis',(-1.,-5.4422705895004E-15,0.));
#14562=DIRECTION('ref_axis',(5.4422705895004E-15,-1.,0.));
#14563=DIRECTION('',(0.,0.,-1.));
#14564=DIRECTION('center_axis',(0.,0.,-1.));
#14565=DIRECTION('ref_axis',(-1.,0.,0.));
#14566=DIRECTION('',(0.,0.,-1.));
#14567=DIRECTION('center_axis',(0.,1.,0.));
#14568=DIRECTION('ref_axis',(0.,0.,1.));
#14569=DIRECTION('',(0.,0.,-1.));
#14570=DIRECTION('center_axis',(0.,0.,-1.));
#14571=DIRECTION('ref_axis',(-1.,0.,0.));
#14572=DIRECTION('',(0.,0.,-1.));
#14573=DIRECTION('center_axis',(-1.,-1.54197609341422E-14,0.));
#14574=DIRECTION('ref_axis',(1.54197609341422E-14,-1.,0.));
#14575=DIRECTION('',(0.,0.,-1.));
#14576=DIRECTION('center_axis',(0.,0.,-1.));
#14577=DIRECTION('ref_axis',(-1.,0.,0.));
#14578=DIRECTION('',(0.,0.,-1.));
#14579=DIRECTION('center_axis',(0.,-1.,0.));
#14580=DIRECTION('ref_axis',(0.,0.,-1.));
#14581=DIRECTION('',(0.,0.,-1.));
#14582=DIRECTION('center_axis',(0.,0.,-1.));
#14583=DIRECTION('ref_axis',(-1.,0.,0.));
#14584=DIRECTION('',(0.,0.,-1.));
#14585=DIRECTION('center_axis',(-1.,0.,0.));
#14586=DIRECTION('ref_axis',(0.,0.,1.));
#14587=DIRECTION('',(0.,0.,-1.));
#14588=DIRECTION('center_axis',(0.,0.,-1.));
#14589=DIRECTION('ref_axis',(-1.,0.,0.));
#14590=DIRECTION('',(0.,0.,-1.));
#14591=DIRECTION('center_axis',(1.68215601615234E-15,-1.,0.));
#14592=DIRECTION('ref_axis',(1.,1.68215601615234E-15,0.));
#14593=DIRECTION('',(0.,0.,-1.));
#14594=DIRECTION('center_axis',(0.,0.,-1.));
#14595=DIRECTION('ref_axis',(-1.,0.,0.));
#14596=DIRECTION('',(0.,0.,-1.));
#14597=DIRECTION('center_axis',(1.,1.68215592970338E-15,0.));
#14598=DIRECTION('ref_axis',(-1.68215592970338E-15,1.,0.));
#14599=DIRECTION('',(0.,0.,-1.));
#14600=DIRECTION('center_axis',(0.,0.,-1.));
#14601=DIRECTION('ref_axis',(-1.,0.,0.));
#14602=DIRECTION('',(0.,0.,-1.));
#14603=DIRECTION('center_axis',(1.38779120854846E-13,1.,0.));
#14604=DIRECTION('ref_axis',(-1.,1.38779120854846E-13,0.));
#14605=DIRECTION('',(0.,0.,-1.));
#14606=DIRECTION('center_axis',(0.,0.,-1.));
#14607=DIRECTION('ref_axis',(-1.,0.,0.));
#14608=DIRECTION('',(0.,0.,-1.));
#14609=DIRECTION('center_axis',(1.,0.,0.));
#14610=DIRECTION('ref_axis',(0.,0.,-1.));
#14611=DIRECTION('',(0.,0.,-1.));
#14612=DIRECTION('center_axis',(0.,0.,-1.));
#14613=DIRECTION('ref_axis',(-1.,0.,0.));
#14614=DIRECTION('',(0.,0.,-1.));
#14615=DIRECTION('center_axis',(-7.70988123297925E-15,1.,0.));
#14616=DIRECTION('ref_axis',(-1.,-7.70988123297925E-15,0.));
#14617=DIRECTION('',(0.,0.,-1.));
#14618=DIRECTION('center_axis',(0.,0.,-1.));
#14619=DIRECTION('ref_axis',(-1.,0.,0.));
#14620=DIRECTION('',(0.,0.,-1.));
#14621=DIRECTION('center_axis',(-1.,-4.0817021727476E-15,0.));
#14622=DIRECTION('ref_axis',(4.0817021727476E-15,-1.,0.));
#14623=DIRECTION('',(0.,0.,-1.));
#14624=DIRECTION('center_axis',(0.,0.,-1.));
#14625=DIRECTION('ref_axis',(-1.,0.,0.));
#14626=DIRECTION('',(0.,0.,-1.));
#14627=DIRECTION('center_axis',(2.72113516754055E-15,1.,0.));
#14628=DIRECTION('ref_axis',(-1.,2.72113516754055E-15,0.));
#14629=DIRECTION('',(0.,0.,-1.));
#14630=DIRECTION('center_axis',(0.707106781186548,0.707106781186548,0.));
#14631=DIRECTION('ref_axis',(-0.707106781186548,0.707106781186548,0.));
#14632=DIRECTION('',(0.,0.,-1.));
#14633=DIRECTION('center_axis',(1.,0.,0.));
#14634=DIRECTION('ref_axis',(0.,0.,-1.));
#14635=DIRECTION('',(0.,0.,-1.));
#14636=DIRECTION('center_axis',(0.866026135466859,0.499998732686731,0.));
#14637=DIRECTION('ref_axis',(-0.499998732686731,0.866026135466859,0.));
#14638=DIRECTION('',(0.,0.,-1.));
#14639=DIRECTION('center_axis',(0.866026135466859,-0.499998732686731,0.));
#14640=DIRECTION('ref_axis',(0.499998732686731,0.866026135466859,0.));
#14641=DIRECTION('',(0.,0.,-1.));
#14642=DIRECTION('center_axis',(1.,0.,0.));
#14643=DIRECTION('ref_axis',(0.,0.,-1.));
#14644=DIRECTION('',(0.,0.,-1.));
#14645=DIRECTION('center_axis',(0.707106781186548,-0.707106781186547,0.));
#14646=DIRECTION('ref_axis',(0.707106781186547,0.707106781186548,0.));
#14647=DIRECTION('',(0.,0.,-1.));
#14648=DIRECTION('center_axis',(0.,-1.,0.));
#14649=DIRECTION('ref_axis',(0.,0.,-1.));
#14650=DIRECTION('',(0.,0.,-1.));
#14651=DIRECTION('center_axis',(0.,0.,-1.));
#14652=DIRECTION('ref_axis',(-1.,0.,0.));
#14653=DIRECTION('',(0.,0.,-1.));
#14654=DIRECTION('center_axis',(-1.,0.,0.));
#14655=DIRECTION('ref_axis',(0.,0.,1.));
#14656=DIRECTION('',(0.,0.,-1.));
#14657=DIRECTION('center_axis',(0.,0.,-1.));
#14658=DIRECTION('ref_axis',(-1.,0.,0.));
#14659=DIRECTION('',(0.,0.,-1.));
#14660=DIRECTION('center_axis',(7.70988123297925E-15,-1.,0.));
#14661=DIRECTION('ref_axis',(1.,7.70988123297925E-15,0.));
#14662=DIRECTION('',(0.,0.,-1.));
#14663=DIRECTION('center_axis',(0.,0.,-1.));
#14664=DIRECTION('ref_axis',(-1.,0.,0.));
#14665=DIRECTION('',(0.,0.,-1.));
#14666=DIRECTION('center_axis',(1.,0.,0.));
#14667=DIRECTION('ref_axis',(0.,0.,-1.));
#14668=DIRECTION('',(0.,0.,-1.));
#14669=DIRECTION('center_axis',(0.,0.,-1.));
#14670=DIRECTION('ref_axis',(-1.,0.,0.));
#14671=DIRECTION('',(0.,0.,-1.));
#14672=DIRECTION('center_axis',(6.93895604274136E-14,-1.,0.));
#14673=DIRECTION('ref_axis',(1.,6.93895604274136E-14,0.));
#14674=DIRECTION('',(0.,0.,-1.));
#14675=DIRECTION('center_axis',(0.,0.,-1.));
#14676=DIRECTION('ref_axis',(-1.,0.,0.));
#14677=DIRECTION('',(0.,0.,-1.));
#14678=DIRECTION('center_axis',(1.,1.68215592970338E-15,0.));
#14679=DIRECTION('ref_axis',(-1.68215592970338E-15,1.,0.));
#14680=DIRECTION('',(0.,0.,-1.));
#14681=DIRECTION('center_axis',(0.,0.,-1.));
#14682=DIRECTION('ref_axis',(-1.,0.,0.));
#14683=DIRECTION('',(0.,0.,-1.));
#14684=DIRECTION('center_axis',(0.,1.,0.));
#14685=DIRECTION('ref_axis',(0.,0.,1.));
#14686=DIRECTION('',(0.,0.,-1.));
#14687=DIRECTION('center_axis',(0.,0.,-1.));
#14688=DIRECTION('ref_axis',(-1.,0.,0.));
#14689=DIRECTION('',(0.,0.,-1.));
#14690=DIRECTION('center_axis',(-1.,0.,0.));
#14691=DIRECTION('ref_axis',(0.,0.,1.));
#14692=DIRECTION('',(0.,0.,-1.));
#14693=DIRECTION('center_axis',(0.,0.,-1.));
#14694=DIRECTION('ref_axis',(-1.,0.,0.));
#14695=DIRECTION('',(0.,0.,-1.));
#14696=DIRECTION('center_axis',(3.46945490866966E-14,1.,0.));
#14697=DIRECTION('ref_axis',(-1.,3.46945490866966E-14,0.));
#14698=DIRECTION('',(0.,0.,-1.));
#14699=DIRECTION('center_axis',(0.,0.,-1.));
#14700=DIRECTION('ref_axis',(-1.,0.,0.));
#14701=DIRECTION('',(0.,0.,-1.));
#14702=DIRECTION('center_axis',(-1.,-1.54197609341422E-14,0.));
#14703=DIRECTION('ref_axis',(1.54197609341422E-14,-1.,0.));
#14704=DIRECTION('',(0.,0.,-1.));
#14705=DIRECTION('center_axis',(0.,0.,-1.));
#14706=DIRECTION('ref_axis',(-1.,0.,0.));
#14707=DIRECTION('',(0.,0.,-1.));
#14708=DIRECTION('center_axis',(-1.0204256560972E-15,-1.,0.));
#14709=DIRECTION('ref_axis',(1.,-1.0204256560972E-15,0.));
#14710=DIRECTION('',(0.,0.,-1.));
#14711=DIRECTION('center_axis',(0.,0.,-1.));
#14712=DIRECTION('ref_axis',(-1.,0.,0.));
#14713=DIRECTION('',(0.,0.,-1.));
#14714=DIRECTION('center_axis',(-1.,0.,0.));
#14715=DIRECTION('ref_axis',(0.,0.,1.));
#14716=DIRECTION('',(0.,0.,-1.));
#14717=DIRECTION('center_axis',(-0.707496679341793,0.706716667923104,0.));
#14718=DIRECTION('ref_axis',(-0.706716667923105,-0.707496679341793,0.));
#14719=DIRECTION('',(0.,0.,-1.));
#14720=DIRECTION('center_axis',(2.09985316358847E-15,1.,0.));
#14721=DIRECTION('ref_axis',(-1.,2.09985316358847E-15,0.));
#14722=DIRECTION('center_axis',(0.,0.,-1.));
#14723=DIRECTION('ref_axis',(0.707106781186544,0.707106781186551,0.));
#14724=DIRECTION('',(0.,0.,-1.));
#14725=DIRECTION('',(0.,0.,-1.));
#14726=DIRECTION('center_axis',(0.,-1.,0.));
#14727=DIRECTION('ref_axis',(0.,0.,-1.));
#14728=DIRECTION('',(0.,0.,-1.));
#14729=DIRECTION('center_axis',(0.,0.,-1.));
#14730=DIRECTION('ref_axis',(-1.,0.,0.));
#14731=DIRECTION('',(0.,0.,-1.));
#14732=DIRECTION('center_axis',(1.,0.,0.));
#14733=DIRECTION('ref_axis',(0.,0.,-1.));
#14734=DIRECTION('',(0.,0.,-1.));
#14735=DIRECTION('center_axis',(0.,0.,-1.));
#14736=DIRECTION('ref_axis',(-1.,0.,0.));
#14737=DIRECTION('',(0.,0.,-1.));
#14738=DIRECTION('center_axis',(-3.15404158980207E-15,1.,0.));
#14739=DIRECTION('ref_axis',(-1.,-3.15404158980207E-15,0.));
#14740=DIRECTION('',(0.,0.,-1.));
#14741=DIRECTION('center_axis',(0.,0.,-1.));
#14742=DIRECTION('ref_axis',(0.707106781186541,-0.707106781186554,0.));
#14743=DIRECTION('',(0.,0.,-1.));
#14744=DIRECTION('center_axis',(-1.,-6.30808317960405E-15,0.));
#14745=DIRECTION('ref_axis',(6.30808317960405E-15,-1.,0.));
#14746=DIRECTION('center_axis',(0.,0.,-1.));
#14747=DIRECTION('ref_axis',(-1.,0.,0.));
#14748=DIRECTION('',(0.,0.,-1.));
#14749=DIRECTION('',(0.,0.,-1.));
#14750=DIRECTION('center_axis',(-0.627534586286487,-0.778588686672397,0.));
#14751=DIRECTION('ref_axis',(0.778588686672397,-0.627534586286487,0.));
#14752=DIRECTION('',(0.,0.,-1.));
#14753=DIRECTION('center_axis',(0.,0.,-1.));
#14754=DIRECTION('ref_axis',(-1.,0.,0.));
#14755=DIRECTION('',(0.,0.,-1.));
#14756=DIRECTION('center_axis',(0.785495070023503,0.61886791399197,0.));
#14757=DIRECTION('ref_axis',(-0.61886791399197,0.785495070023503,0.));
#14758=DIRECTION('center_axis',(0.785495070023487,-0.61886791399199,0.));
#14759=DIRECTION('ref_axis',(0.61886791399199,0.785495070023487,0.));
#14760=DIRECTION('',(0.,0.,-1.));
#14761=DIRECTION('center_axis',(0.,0.,-1.));
#14762=DIRECTION('ref_axis',(-1.,0.,0.));
#14763=DIRECTION('',(0.,0.,-1.));
#14764=DIRECTION('center_axis',(-0.627534586286517,0.778588686672372,0.));
#14765=DIRECTION('ref_axis',(-0.778588686672372,-0.627534586286517,0.));
#14766=DIRECTION('',(0.,0.,-1.));
#14767=DIRECTION('center_axis',(0.,0.,-1.));
#14768=DIRECTION('ref_axis',(-1.,0.,0.));
#14769=DIRECTION('',(0.,0.,-1.));
#14770=DIRECTION('center_axis',(0.627534586286505,0.778588686672382,0.));
#14771=DIRECTION('ref_axis',(-0.778588686672382,0.627534586286505,0.));
#14772=DIRECTION('',(0.,0.,-1.));
#14773=DIRECTION('center_axis',(0.,0.,-1.));
#14774=DIRECTION('ref_axis',(-1.,0.,0.));
#14775=DIRECTION('',(0.,0.,-1.));
#14776=DIRECTION('center_axis',(-0.785495070023481,-0.618867913991998,0.));
#14777=DIRECTION('ref_axis',(0.618867913991998,-0.785495070023481,0.));
#14778=DIRECTION('',(0.,0.,-1.));
#14779=DIRECTION('center_axis',(0.,0.,-1.));
#14780=DIRECTION('ref_axis',(1.,-3.21624529935327E-16,0.));
#14781=DIRECTION('',(0.,0.,-1.));
#14782=DIRECTION('center_axis',(-0.785495070023503,0.61886791399197,0.));
#14783=DIRECTION('ref_axis',(-0.61886791399197,-0.785495070023503,0.));
#14784=DIRECTION('',(0.,0.,-1.));
#14785=DIRECTION('center_axis',(0.,0.,-1.));
#14786=DIRECTION('ref_axis',(-1.,0.,0.));
#14787=DIRECTION('',(0.,0.,-1.));
#14788=DIRECTION('center_axis',(0.627534586286492,-0.778588686672393,0.));
#14789=DIRECTION('ref_axis',(0.778588686672393,0.627534586286492,0.));
#14790=DIRECTION('center_axis',(0.,0.,-1.));
#14791=DIRECTION('ref_axis',(-1.,0.,0.));
#14792=DIRECTION('',(0.,0.,-1.));
#14793=DIRECTION('',(0.,0.,-1.));
#14794=DIRECTION('center_axis',(0.,1.,0.));
#14795=DIRECTION('ref_axis',(0.,0.,1.));
#14796=DIRECTION('',(0.,0.,-1.));
#14797=DIRECTION('center_axis',(0.,0.,-1.));
#14798=DIRECTION('ref_axis',(0.707106781186549,-0.707106781186546,0.));
#14799=DIRECTION('',(0.,0.,-1.));
#14800=DIRECTION('center_axis',(-1.,0.,0.));
#14801=DIRECTION('ref_axis',(0.,0.,1.));
#14802=DIRECTION('',(0.,0.,-1.));
#14803=DIRECTION('center_axis',(0.,0.,-1.));
#14804=DIRECTION('ref_axis',(0.707106781186547,0.707106781186548,0.));
#14805=DIRECTION('',(0.,0.,-1.));
#14806=DIRECTION('center_axis',(3.15404158980205E-15,-1.,0.));
#14807=DIRECTION('ref_axis',(1.,3.15404158980205E-15,0.));
#14808=DIRECTION('',(0.,0.,-1.));
#14809=DIRECTION('center_axis',(0.,0.,-1.));
#14810=DIRECTION('ref_axis',(-1.,0.,0.));
#14811=DIRECTION('',(0.,0.,-1.));
#14812=DIRECTION('center_axis',(1.,6.30808317960409E-15,0.));
#14813=DIRECTION('ref_axis',(-6.30808317960409E-15,1.,0.));
#14814=DIRECTION('center_axis',(0.,0.,-1.));
#14815=DIRECTION('ref_axis',(0.707106781186549,-0.707106781186546,0.));
#14816=DIRECTION('',(0.,0.,-1.));
#14817=DIRECTION('',(0.,0.,-1.));
#14818=DIRECTION('center_axis',(-1.,-6.30808317960404E-15,0.));
#14819=DIRECTION('ref_axis',(6.30808317960404E-15,-1.,0.));
#14820=DIRECTION('',(0.,0.,-1.));
#14821=DIRECTION('center_axis',(0.,0.,-1.));
#14822=DIRECTION('ref_axis',(0.707106781186541,0.707106781186554,0.));
#14823=DIRECTION('',(0.,0.,-1.));
#14824=DIRECTION('center_axis',(0.,-1.,0.));
#14825=DIRECTION('ref_axis',(0.,0.,-1.));
#14826=DIRECTION('',(0.,0.,-1.));
#14827=DIRECTION('center_axis',(0.,0.,-1.));
#14828=DIRECTION('ref_axis',(-1.,0.,0.));
#14829=DIRECTION('',(0.,0.,-1.));
#14830=DIRECTION('center_axis',(1.,0.,0.));
#14831=DIRECTION('ref_axis',(0.,0.,-1.));
#14832=DIRECTION('',(0.,0.,-1.));
#14833=DIRECTION('center_axis',(0.,0.,-1.));
#14834=DIRECTION('ref_axis',(-1.,0.,0.));
#14835=DIRECTION('',(0.,0.,-1.));
#14836=DIRECTION('center_axis',(-3.15404158980205E-15,1.,0.));
#14837=DIRECTION('ref_axis',(-1.,-3.15404158980205E-15,0.));
#14838=DIRECTION('center_axis',(0.,0.,-1.));
#14839=DIRECTION('ref_axis',(0.707106781186551,0.707106781186544,0.));
#14840=DIRECTION('',(0.,0.,-1.));
#14841=DIRECTION('',(0.,0.,-1.));
#14842=DIRECTION('center_axis',(0.,-1.,0.));
#14843=DIRECTION('ref_axis',(0.,0.,-1.));
#14844=DIRECTION('',(0.,0.,-1.));
#14845=DIRECTION('center_axis',(0.,0.,-1.));
#14846=DIRECTION('ref_axis',(-1.,0.,0.));
#14847=DIRECTION('',(0.,0.,-1.));
#14848=DIRECTION('center_axis',(1.,6.30808317960409E-15,0.));
#14849=DIRECTION('ref_axis',(-6.30808317960409E-15,1.,0.));
#14850=DIRECTION('',(0.,0.,-1.));
#14851=DIRECTION('center_axis',(0.,0.,-1.));
#14852=DIRECTION('ref_axis',(-1.,0.,0.));
#14853=DIRECTION('',(0.,0.,-1.));
#14854=DIRECTION('center_axis',(0.,1.,0.));
#14855=DIRECTION('ref_axis',(0.,0.,1.));
#14856=DIRECTION('',(0.,0.,-1.));
#14857=DIRECTION('center_axis',(0.,0.,-1.));
#14858=DIRECTION('ref_axis',(0.707106781186548,-0.707106781186547,0.));
#14859=DIRECTION('',(0.,0.,-1.));
#14860=DIRECTION('center_axis',(-1.,0.,0.));
#14861=DIRECTION('ref_axis',(0.,0.,1.));
#17191=CARTESIAN_POINT('',(0.,0.,0.));
#17192=CARTESIAN_POINT('Origin',(96.5599999999999,35.0599999999999,380.));
#17193=CARTESIAN_POINT('',(93.2794382684679,36.6601295965039,380.));
#17194=CARTESIAN_POINT('',(93.279438268468,33.4598704034959,380.));
#17195=CARTESIAN_POINT('Origin',(96.5599999999999,35.0599999999999,380.));
#17196=CARTESIAN_POINT('',(93.279438268468,33.4598704034959,0.));
#17197=CARTESIAN_POINT('',(93.279438268468,33.4598704034959,380.));
#17198=CARTESIAN_POINT('',(93.2794382684679,36.6601295965039,0.));
#17199=CARTESIAN_POINT('Origin',(96.5599999999999,35.0599999999999,0.));
#17200=CARTESIAN_POINT('',(93.2794382684679,36.6601295965039,380.));
#17201=CARTESIAN_POINT('Origin',(104.609999923724,22.4600011663401,380.));
#17202=CARTESIAN_POINT('',(95.6600000543452,29.0599999999999,380.));
#17203=CARTESIAN_POINT('',(96.5599999999999,29.5751481628425,380.));
#17204=CARTESIAN_POINT('',(95.6600000543452,29.0599999999999,380.));
#17205=CARTESIAN_POINT('',(97.4599999456547,29.0599999999999,380.));
#17206=CARTESIAN_POINT('',(96.5599999999999,29.5751481628425,380.));
#17207=CARTESIAN_POINT('',(100.764466193213,29.0599999999999,380.));
#17208=CARTESIAN_POINT('',(97.4599999456547,29.0599999999999,380.));
#17209=CARTESIAN_POINT('',(104.810000327124,25.0100007629401,380.));
#17210=CARTESIAN_POINT('',(100.764466193213,29.0599999999999,380.));
#17211=CARTESIAN_POINT('',(104.810000327124,22.4600011663401,380.));
#17212=CARTESIAN_POINT('',(104.810000327124,25.0100007629401,380.));
#17213=CARTESIAN_POINT('',(104.609999923724,22.2600007629398,380.));
#17214=CARTESIAN_POINT('Origin',(104.609999923724,22.4600011663401,380.));
#17215=CARTESIAN_POINT('',(101.210000196921,22.2600007629398,380.));
#17216=CARTESIAN_POINT('',(104.609999923724,22.2600007629398,380.));
#17217=CARTESIAN_POINT('',(100.61,21.6600005660189,380.));
#17218=CARTESIAN_POINT('Origin',(101.210000196921,21.6600005660189,380.));
#17219=CARTESIAN_POINT('',(100.61,20.7600003735979,380.));
#17220=CARTESIAN_POINT('',(100.61,21.6600005660189,380.));
#17221=CARTESIAN_POINT('',(100.810000373598,20.5599999999999,380.));
#17222=CARTESIAN_POINT('Origin',(100.810000373598,20.7600003735979,380.));
#17223=CARTESIAN_POINT('',(100.910000144262,20.5599999999999,380.));
#17224=CARTESIAN_POINT('',(100.810000373598,20.5599999999999,380.));
#17225=CARTESIAN_POINT('',(101.109999564186,20.3600005800758,380.));
#17226=CARTESIAN_POINT('Origin',(100.910000144262,20.3600005800758,380.));
#17227=CARTESIAN_POINT('',(101.109999564186,20.2600003810484,380.));
#17228=CARTESIAN_POINT('',(101.109999564186,20.3600005800758,380.));
#17229=CARTESIAN_POINT('',(101.309999945234,20.0599999999999,380.));
#17230=CARTESIAN_POINT('Origin',(101.309999945234,20.2600003810484,380.));
#17231=CARTESIAN_POINT('',(109.560000346242,20.0599999999999,380.));
#17232=CARTESIAN_POINT('',(101.309999945234,20.0599999999999,380.));
#17233=CARTESIAN_POINT('',(111.56,22.0599996537577,380.));
#17234=CARTESIAN_POINT('Origin',(109.560000346242,22.0599996537577,380.));
#17235=CARTESIAN_POINT('',(111.56,30.3100004787476,380.));
#17236=CARTESIAN_POINT('',(111.56,22.0599996537577,380.));
#17237=CARTESIAN_POINT('',(111.359999715809,30.5100007629388,380.));
#17238=CARTESIAN_POINT('Origin',(111.359999715809,30.3100004787476,380.));
#17239=CARTESIAN_POINT('',(111.260000611316,30.5100007629388,380.));
#17240=CARTESIAN_POINT('',(111.359999715809,30.5100007629388,380.));
#17241=CARTESIAN_POINT('',(111.060000327124,30.71000104713,380.));
#17242=CARTESIAN_POINT('Origin',(111.260000611316,30.71000104713,380.));
#17243=CARTESIAN_POINT('',(111.060000327124,30.8100004787487,380.));
#17244=CARTESIAN_POINT('',(111.060000327124,30.71000104713,380.));
#17245=CARTESIAN_POINT('',(110.860000042933,31.0100007629399,380.));
#17246=CARTESIAN_POINT('Origin',(110.860000042933,30.8100004787487,380.));
#17247=CARTESIAN_POINT('',(109.959999939919,31.0100007629399,380.));
#17248=CARTESIAN_POINT('',(110.860000042933,31.0100007629399,380.));
#17249=CARTESIAN_POINT('',(109.359999564184,30.4100003872052,380.));
#17250=CARTESIAN_POINT('Origin',(109.959999939919,30.4100003872052,380.));
#17251=CARTESIAN_POINT('',(109.359999564184,27.0100002841911,380.));
#17252=CARTESIAN_POINT('',(109.359999564184,30.4100003872052,380.));
#17253=CARTESIAN_POINT('',(109.159999279993,26.8099999999999,380.));
#17254=CARTESIAN_POINT('Origin',(109.159999279993,27.0100002841911,380.));
#17255=CARTESIAN_POINT('',(106.609999564184,26.8099999999999,380.));
#17256=CARTESIAN_POINT('',(109.159999279993,26.8099999999999,380.));
#17257=CARTESIAN_POINT('',(102.564465430273,30.8555341339111,380.));
#17258=CARTESIAN_POINT('',(106.609999564184,26.8099999999999,380.));
#17259=CARTESIAN_POINT('',(102.564465430273,34.1600003814696,380.));
#17260=CARTESIAN_POINT('',(102.564465430273,30.8555341339111,380.));
#17261=CARTESIAN_POINT('',(102.044852164282,35.0599999999999,380.));
#17262=CARTESIAN_POINT('',(102.564465430273,34.1600003814696,380.));
#17263=CARTESIAN_POINT('',(102.564465430273,35.9599996185302,380.));
#17264=CARTESIAN_POINT('',(102.044852164282,35.0599999999999,380.));
#17265=CARTESIAN_POINT('',(102.564465430273,39.2644658660888,380.));
#17266=CARTESIAN_POINT('',(102.564465430273,35.9599996185302,380.));
#17267=CARTESIAN_POINT('',(106.609999564184,43.3099999999999,380.));
#17268=CARTESIAN_POINT('',(102.564465430273,39.2644658660888,380.));
#17269=CARTESIAN_POINT('',(109.159999279993,43.3099999999999,380.));
#17270=CARTESIAN_POINT('',(106.609999564184,43.3099999999999,380.));
#17271=CARTESIAN_POINT('',(109.359999564184,43.1099997158087,380.));
#17272=CARTESIAN_POINT('Origin',(109.159999279993,43.1099997158087,380.));
#17273=CARTESIAN_POINT('',(109.359999564184,39.7099996127947,380.));
#17274=CARTESIAN_POINT('',(109.359999564184,43.1099997158087,380.));
#17275=CARTESIAN_POINT('',(109.959999939919,39.1099992370599,380.));
#17276=CARTESIAN_POINT('Origin',(109.959999939919,39.7099996127947,380.));
#17277=CARTESIAN_POINT('',(110.860000042933,39.1099992370599,380.));
#17278=CARTESIAN_POINT('',(109.959999939919,39.1099992370599,380.));
#17279=CARTESIAN_POINT('',(111.060000327124,39.3099995212511,380.));
#17280=CARTESIAN_POINT('Origin',(110.860000042933,39.3099995212511,380.));
#17281=CARTESIAN_POINT('',(111.060000327124,39.4099989528698,380.));
#17282=CARTESIAN_POINT('',(111.060000327124,39.3099995212511,380.));
#17283=CARTESIAN_POINT('',(111.260000611316,39.609999237061,380.));
#17284=CARTESIAN_POINT('Origin',(111.260000611316,39.4099989528698,380.));
#17285=CARTESIAN_POINT('',(111.359999715809,39.609999237061,380.));
#17286=CARTESIAN_POINT('',(111.260000611316,39.609999237061,380.));
#17287=CARTESIAN_POINT('',(111.56,39.8099995212523,380.));
#17288=CARTESIAN_POINT('Origin',(111.359999715809,39.8099995212523,380.));
#17289=CARTESIAN_POINT('',(111.56,48.0600003462421,380.));
#17290=CARTESIAN_POINT('',(111.56,39.8099995212523,380.));
#17291=CARTESIAN_POINT('',(109.560000346242,50.0599999999999,380.));
#17292=CARTESIAN_POINT('Origin',(109.560000346242,48.0600003462421,380.));
#17293=CARTESIAN_POINT('',(101.309999945234,50.0599999999999,380.));
#17294=CARTESIAN_POINT('',(109.560000346242,50.0599999999999,380.));
#17295=CARTESIAN_POINT('',(101.109999564186,49.8599996189514,380.));
#17296=CARTESIAN_POINT('Origin',(101.309999945234,49.8599996189514,380.));
#17297=CARTESIAN_POINT('',(101.109999564186,49.759999419924,380.));
#17298=CARTESIAN_POINT('',(101.109999564186,49.8599996189514,380.));
#17299=CARTESIAN_POINT('',(100.910000144262,49.5599999999999,380.));
#17300=CARTESIAN_POINT('Origin',(100.910000144262,49.759999419924,380.));
#17301=CARTESIAN_POINT('',(100.810000373598,49.5599999999999,380.));
#17302=CARTESIAN_POINT('',(100.910000144262,49.5599999999999,380.));
#17303=CARTESIAN_POINT('',(100.61,49.3599996264019,380.));
#17304=CARTESIAN_POINT('Origin',(100.810000373598,49.3599996264019,380.));
#17305=CARTESIAN_POINT('',(100.61,48.4599994339809,380.));
#17306=CARTESIAN_POINT('',(100.61,49.3599996264019,380.));
#17307=CARTESIAN_POINT('',(101.210000196921,47.85999923706,380.));
#17308=CARTESIAN_POINT('Origin',(101.210000196921,48.4599994339809,380.));
#17309=CARTESIAN_POINT('',(104.609999923724,47.85999923706,380.));
#17310=CARTESIAN_POINT('',(101.210000196921,47.85999923706,380.));
#17311=CARTESIAN_POINT('',(104.810000327124,47.6599988336597,380.));
#17312=CARTESIAN_POINT('Origin',(104.609999923724,47.6599988336597,380.));
#17313=CARTESIAN_POINT('',(104.810000327124,45.1099992370597,380.));
#17314=CARTESIAN_POINT('',(104.810000327124,47.6599988336597,380.));
#17315=CARTESIAN_POINT('',(100.764466193213,41.0599999999999,380.));
#17316=CARTESIAN_POINT('',(104.810000327124,45.1099992370597,380.));
#17317=CARTESIAN_POINT('',(97.4599999456547,41.0599999999999,380.));
#17318=CARTESIAN_POINT('',(100.764466193213,41.0599999999999,380.));
#17319=CARTESIAN_POINT('',(96.5599999999999,40.5448518371574,380.));
#17320=CARTESIAN_POINT('',(97.4599999456547,41.0599999999999,380.));
#17321=CARTESIAN_POINT('',(95.6600000543452,41.0599999999999,380.));
#17322=CARTESIAN_POINT('',(96.5599999999999,40.5448518371574,380.));
#17323=CARTESIAN_POINT('',(92.3555338067866,41.0599999999999,380.));
#17324=CARTESIAN_POINT('',(95.6600000543452,41.0599999999999,380.));
#17325=CARTESIAN_POINT('',(88.3099996728755,45.1099992370597,380.));
#17326=CARTESIAN_POINT('',(92.3555338067866,41.0599999999999,380.));
#17327=CARTESIAN_POINT('',(88.3099996728755,47.6599988336597,380.));
#17328=CARTESIAN_POINT('',(88.3099996728755,45.1099992370597,380.));
#17329=CARTESIAN_POINT('',(88.5100000762757,47.85999923706,380.));
#17330=CARTESIAN_POINT('Origin',(88.5100000762757,47.6599988336597,380.));
#17331=CARTESIAN_POINT('',(91.9099998030791,47.85999923706,380.));
#17332=CARTESIAN_POINT('',(88.5100000762757,47.85999923706,380.));
#17333=CARTESIAN_POINT('',(92.5099999999999,48.4599994339809,380.));
#17334=CARTESIAN_POINT('Origin',(91.9099998030791,48.4599994339809,380.));
#17335=CARTESIAN_POINT('',(92.5099999999999,49.3599996264019,380.));
#17336=CARTESIAN_POINT('',(92.5099999999999,48.4599994339809,380.));
#17337=CARTESIAN_POINT('',(92.309999626402,49.5599999999999,380.));
#17338=CARTESIAN_POINT('Origin',(92.309999626402,49.3599996264019,380.));
#17339=CARTESIAN_POINT('',(92.2099998557381,49.5599999999999,380.));
#17340=CARTESIAN_POINT('',(92.309999626402,49.5599999999999,380.));
#17341=CARTESIAN_POINT('',(92.010000435814,49.759999419924,380.));
#17342=CARTESIAN_POINT('Origin',(92.2099998557381,49.759999419924,380.));
#17343=CARTESIAN_POINT('',(92.010000435814,49.8599996189514,380.));
#17344=CARTESIAN_POINT('',(92.010000435814,49.759999419924,380.));
#17345=CARTESIAN_POINT('',(91.8100000547655,50.0599999999999,380.));
#17346=CARTESIAN_POINT('Origin',(91.8100000547655,49.8599996189514,380.));
#17347=CARTESIAN_POINT('',(83.5599996537577,50.0599999999999,380.));
#17348=CARTESIAN_POINT('',(91.8100000547655,50.0599999999999,380.));
#17349=CARTESIAN_POINT('',(81.5599999999999,48.0600003462421,380.));
#17350=CARTESIAN_POINT('Origin',(83.5599996537577,48.0600003462421,380.));
#17351=CARTESIAN_POINT('',(81.5599999999999,39.8099995212522,380.));
#17352=CARTESIAN_POINT('',(81.5599999999999,48.0600003462421,380.));
#17353=CARTESIAN_POINT('',(81.7600002841911,39.609999237061,380.));
#17354=CARTESIAN_POINT('Origin',(81.7600002841911,39.8099995212522,380.));
#17355=CARTESIAN_POINT('',(81.8599993886842,39.609999237061,380.));
#17356=CARTESIAN_POINT('',(81.7600002841911,39.609999237061,380.));
#17357=CARTESIAN_POINT('',(82.0599996728754,39.4099989528698,380.));
#17358=CARTESIAN_POINT('Origin',(81.8599993886842,39.4099989528698,380.));
#17359=CARTESIAN_POINT('',(82.0599996728754,39.3099995212511,380.));
#17360=CARTESIAN_POINT('',(82.0599996728754,39.4099989528698,380.));
#17361=CARTESIAN_POINT('',(82.2599999570666,39.1099992370599,380.));
#17362=CARTESIAN_POINT('Origin',(82.2599999570666,39.3099995212511,380.));
#17363=CARTESIAN_POINT('',(83.1600000600806,39.1099992370599,380.));
#17364=CARTESIAN_POINT('',(82.2599999570666,39.1099992370599,380.));
#17365=CARTESIAN_POINT('',(83.7600004358154,39.7099996127947,380.));
#17366=CARTESIAN_POINT('Origin',(83.1600000600806,39.7099996127947,380.));
#17367=CARTESIAN_POINT('',(83.7600004358154,43.1099997158087,380.));
#17368=CARTESIAN_POINT('',(83.7600004358154,39.7099996127947,380.));
#17369=CARTESIAN_POINT('',(83.9600007200066,43.3099999999999,380.));
#17370=CARTESIAN_POINT('Origin',(83.9600007200066,43.1099997158087,380.));
#17371=CARTESIAN_POINT('',(86.510000435816,43.3099999999999,380.));
#17372=CARTESIAN_POINT('',(83.9600007200066,43.3099999999999,380.));
#17373=CARTESIAN_POINT('',(90.5555345697271,39.2644658660888,380.));
#17374=CARTESIAN_POINT('',(86.510000435816,43.3099999999999,380.));
#17375=CARTESIAN_POINT('',(90.5555345697271,35.9599996185302,380.));
#17376=CARTESIAN_POINT('',(90.5555345697271,39.2644658660888,380.));
#17377=CARTESIAN_POINT('',(91.0751478357183,35.0599999999999,380.));
#17378=CARTESIAN_POINT('',(90.5555345697271,35.9599996185302,380.));
#17379=CARTESIAN_POINT('',(90.5555345697271,34.1600003814696,380.));
#17380=CARTESIAN_POINT('',(91.0751478357183,35.0599999999999,380.));
#17381=CARTESIAN_POINT('',(90.5555345697271,30.8555341339111,380.));
#17382=CARTESIAN_POINT('',(90.5555345697271,34.1600003814696,380.));
#17383=CARTESIAN_POINT('',(86.510000435816,26.8099999999999,380.));
#17384=CARTESIAN_POINT('',(90.5555345697271,30.8555341339111,380.));
#17385=CARTESIAN_POINT('',(83.9600007200066,26.8099999999999,380.));
#17386=CARTESIAN_POINT('',(86.510000435816,26.8099999999999,380.));
#17387=CARTESIAN_POINT('',(83.7600004358154,27.0100002841911,380.));
#17388=CARTESIAN_POINT('Origin',(83.9600007200066,27.0100002841911,380.));
#17389=CARTESIAN_POINT('',(83.7600004358154,30.4100003872052,380.));
#17390=CARTESIAN_POINT('',(83.7600004358154,27.0100002841911,380.));
#17391=CARTESIAN_POINT('',(83.1600000600806,31.0100007629399,380.));
#17392=CARTESIAN_POINT('Origin',(83.1600000600806,30.4100003872052,380.));
#17393=CARTESIAN_POINT('',(82.2599999570666,31.0100007629399,380.));
#17394=CARTESIAN_POINT('',(83.1600000600806,31.0100007629399,380.));
#17395=CARTESIAN_POINT('',(82.0599996728754,30.8100004787487,380.));
#17396=CARTESIAN_POINT('Origin',(82.2599999570666,30.8100004787487,380.));
#17397=CARTESIAN_POINT('',(82.0599996728754,30.71000104713,380.));
#17398=CARTESIAN_POINT('',(82.0599996728754,30.8100004787487,380.));
#17399=CARTESIAN_POINT('',(81.8599993886842,30.5100007629388,380.));
#17400=CARTESIAN_POINT('Origin',(81.8599993886842,30.71000104713,380.));
#17401=CARTESIAN_POINT('',(81.7600002841911,30.5100007629388,380.));
#17402=CARTESIAN_POINT('',(81.8599993886842,30.5100007629388,380.));
#17403=CARTESIAN_POINT('',(81.5599999999999,30.3100004787476,380.));
#17404=CARTESIAN_POINT('Origin',(81.7600002841911,30.3100004787476,380.));
#17405=CARTESIAN_POINT('',(81.5599999999999,22.0599996537577,380.));
#17406=CARTESIAN_POINT('',(81.5599999999999,30.3100004787476,380.));
#17407=CARTESIAN_POINT('',(83.5599996537578,20.0599999999999,380.));
#17408=CARTESIAN_POINT('Origin',(83.5599996537577,22.0599996537577,380.));
#17409=CARTESIAN_POINT('',(91.8100000547655,20.0599999999999,380.));
#17410=CARTESIAN_POINT('',(83.5599996537578,20.0599999999999,380.));
#17411=CARTESIAN_POINT('',(92.010000435814,20.2600003810484,380.));
#17412=CARTESIAN_POINT('Origin',(91.8100000547655,20.2600003810484,380.));
#17413=CARTESIAN_POINT('',(92.010000435814,20.3600005800758,380.));
#17414=CARTESIAN_POINT('',(92.010000435814,20.2600003810484,380.));
#17415=CARTESIAN_POINT('',(92.2099998557381,20.5599999999999,380.));
#17416=CARTESIAN_POINT('Origin',(92.2099998557381,20.3600005800758,380.));
#17417=CARTESIAN_POINT('',(92.309999626402,20.5599999999999,380.));
#17418=CARTESIAN_POINT('',(92.2099998557381,20.5599999999999,380.));
#17419=CARTESIAN_POINT('',(92.5099999999999,20.7600003735979,380.));
#17420=CARTESIAN_POINT('Origin',(92.309999626402,20.7600003735979,380.));
#17421=CARTESIAN_POINT('',(92.5099999999999,21.6600005660189,380.));
#17422=CARTESIAN_POINT('',(92.5099999999999,20.7600003735979,380.));
#17423=CARTESIAN_POINT('',(91.9099998030791,22.2600007629398,380.));
#17424=CARTESIAN_POINT('Origin',(91.9099998030791,21.6600005660189,380.));
#17425=CARTESIAN_POINT('',(88.5100000762757,22.2600007629398,380.));
#17426=CARTESIAN_POINT('',(91.9099998030791,22.2600007629398,380.));
#17427=CARTESIAN_POINT('',(88.3099996728755,22.4600011663401,380.));
#17428=CARTESIAN_POINT('Origin',(88.5100000762757,22.4600011663401,380.));
#17429=CARTESIAN_POINT('',(88.3099996728755,25.0100007629401,380.));
#17430=CARTESIAN_POINT('',(88.3099996728755,22.4600011663401,380.));
#17431=CARTESIAN_POINT('',(92.3555338067866,29.0599999999999,380.));
#17432=CARTESIAN_POINT('',(88.3099996728755,25.0100007629401,380.));
#17433=CARTESIAN_POINT('',(92.3555338067866,29.0599999999999,380.));
#17434=CARTESIAN_POINT('',(109.260001090064,48.7600003984092,380.));
#17435=CARTESIAN_POINT('',(107.060000327124,48.7600003984092,380.));
#17436=CARTESIAN_POINT('',(109.260001090064,48.7600003984092,380.));
#17437=CARTESIAN_POINT('',(110.260001090064,47.7600003984092,380.));
#17438=CARTESIAN_POINT('Origin',(109.260001099622,47.7600004079674,380.));
#17439=CARTESIAN_POINT('',(110.260001090064,45.5599996354697,380.));
#17440=CARTESIAN_POINT('',(110.260001090064,45.5599996354697,380.));
#17441=CARTESIAN_POINT('',(109.260001090064,44.5599996354697,380.));
#17442=CARTESIAN_POINT('Origin',(109.260001099622,45.5599996259115,380.));
#17443=CARTESIAN_POINT('',(107.060000327124,44.5599996354697,380.));
#17444=CARTESIAN_POINT('',(107.060000327124,44.5599996354697,380.));
#17445=CARTESIAN_POINT('',(106.060000327124,45.5599996354697,380.));
#17446=CARTESIAN_POINT('Origin',(107.060000317566,45.5599996259115,380.));
#17447=CARTESIAN_POINT('',(106.060000327124,47.7600003984092,380.));
#17448=CARTESIAN_POINT('',(106.060000327124,47.7600003984092,380.));
#17449=CARTESIAN_POINT('Origin',(107.060000317566,47.7600004079674,380.));
#17450=CARTESIAN_POINT('',(94.9598704761907,38.3405617669895,380.));
#17451=CARTESIAN_POINT('',(93.4240705880017,39.5784009033024,380.));
#17452=CARTESIAN_POINT('',(94.9598704761907,38.3405617669895,380.));
#17453=CARTESIAN_POINT('',(98.1601295238092,38.3405617669895,380.));
#17454=CARTESIAN_POINT('Origin',(96.5599999999999,35.0599999999999,380.));
#17455=CARTESIAN_POINT('',(99.6959294119981,39.5784009033024,380.));
#17456=CARTESIAN_POINT('',(99.6959294119981,39.5784009033024,380.));
#17457=CARTESIAN_POINT('',(101.065336892425,38.2146694732975,380.));
#17458=CARTESIAN_POINT('Origin',(96.5599999999999,35.0599999999999,380.));
#17459=CARTESIAN_POINT('',(99.8405617315319,36.6601295965039,380.));
#17460=CARTESIAN_POINT('',(99.8405617315319,36.6601295965039,380.));
#17461=CARTESIAN_POINT('',(99.8405617315319,33.459870403496,380.));
#17462=CARTESIAN_POINT('Origin',(96.5599999999999,35.0599999999999,380.));
#17463=CARTESIAN_POINT('',(101.065336892425,31.9053305267024,380.));
#17464=CARTESIAN_POINT('',(101.065336892425,31.9053305267024,380.));
#17465=CARTESIAN_POINT('',(99.6959294119981,30.5415990966974,380.));
#17466=CARTESIAN_POINT('Origin',(96.5599999999999,35.0599999999999,380.));
#17467=CARTESIAN_POINT('',(98.1601295238092,31.7794382330103,380.));
#17468=CARTESIAN_POINT('',(98.1601295238092,31.7794382330103,380.));
#17469=CARTESIAN_POINT('',(94.9598704761907,31.7794382330103,380.));
#17470=CARTESIAN_POINT('Origin',(96.5599999999999,35.0599999999999,380.));
#17471=CARTESIAN_POINT('',(93.4240705880018,30.5415990966974,380.));
#17472=CARTESIAN_POINT('',(93.4240705880018,30.5415990966974,380.));
#17473=CARTESIAN_POINT('',(92.0546631075751,31.9053305267024,380.));
#17474=CARTESIAN_POINT('Origin',(96.5599999999999,35.0599999999999,380.));
#17475=CARTESIAN_POINT('',(93.279438268468,33.4598704034959,380.));
#17476=CARTESIAN_POINT('',(92.0546631075751,38.2146694732975,380.));
#17477=CARTESIAN_POINT('',(92.0546631075751,38.2146694732975,380.));
#17478=CARTESIAN_POINT('Origin',(96.5599999999999,35.0599999999999,380.));
#17479=CARTESIAN_POINT('',(83.859998909936,21.3599996015906,380.));
#17480=CARTESIAN_POINT('',(86.0599996728755,21.3599996015906,380.));
#17481=CARTESIAN_POINT('',(83.859998909936,21.3599996015906,380.));
#17482=CARTESIAN_POINT('',(82.8599989099361,22.3599996015906,380.));
#17483=CARTESIAN_POINT('Origin',(83.8599989003778,22.3599995920324,380.));
#17484=CARTESIAN_POINT('',(82.859998909936,24.5600003645301,380.));
#17485=CARTESIAN_POINT('',(82.859998909936,24.5600003645301,380.));
#17486=CARTESIAN_POINT('',(83.859998909936,25.5600003645301,380.));
#17487=CARTESIAN_POINT('Origin',(83.8599989003778,24.5600003740883,380.));
#17488=CARTESIAN_POINT('',(86.0599996728755,25.5600003645301,380.));
#17489=CARTESIAN_POINT('',(86.0599996728755,25.5600003645301,380.));
#17490=CARTESIAN_POINT('',(87.0599996728755,24.5600003645301,380.));
#17491=CARTESIAN_POINT('Origin',(86.0599996824337,24.5600003740883,380.));
#17492=CARTESIAN_POINT('',(87.0599996728755,22.3599996015906,380.));
#17493=CARTESIAN_POINT('',(87.0599996728755,22.3599996015906,380.));
#17494=CARTESIAN_POINT('Origin',(86.0599996824337,22.3599995920324,380.));
#17495=CARTESIAN_POINT('',(110.260001090064,22.3599996015906,380.));
#17496=CARTESIAN_POINT('',(110.260001090064,24.5600003645301,380.));
#17497=CARTESIAN_POINT('',(110.260001090064,22.3599996015906,380.));
#17498=CARTESIAN_POINT('',(109.260001090064,21.3599996015906,380.));
#17499=CARTESIAN_POINT('Origin',(109.260001099622,22.3599995920324,380.));
#17500=CARTESIAN_POINT('',(107.060000327124,21.3599996015906,380.));
#17501=CARTESIAN_POINT('',(107.060000327124,21.3599996015906,380.));
#17502=CARTESIAN_POINT('',(106.060000327124,22.3599996015906,380.));
#17503=CARTESIAN_POINT('Origin',(107.060000317566,22.3599995920324,380.));
#17504=CARTESIAN_POINT('',(106.060000327124,24.5600003645301,380.));
#17505=CARTESIAN_POINT('',(106.060000327124,24.5600003645301,380.));
#17506=CARTESIAN_POINT('',(107.060000327124,25.5600003645301,380.));
#17507=CARTESIAN_POINT('Origin',(107.060000317566,24.5600003740883,380.));
#17508=CARTESIAN_POINT('',(109.260001090064,25.5600003645301,380.));
#17509=CARTESIAN_POINT('',(109.260001090064,25.5600003645301,380.));
#17510=CARTESIAN_POINT('Origin',(109.260001099622,24.5600003740883,380.));
#17511=CARTESIAN_POINT('',(86.0599996728755,48.7600003984092,380.));
#17512=CARTESIAN_POINT('',(83.859998909936,48.7600003984092,380.));
#17513=CARTESIAN_POINT('',(86.0599996728755,48.7600003984092,380.));
#17514=CARTESIAN_POINT('',(87.0599996728755,47.7600003984092,380.));
#17515=CARTESIAN_POINT('Origin',(86.0599996824337,47.7600004079674,380.));
#17516=CARTESIAN_POINT('',(87.0599996728755,45.5599996354697,380.));
#17517=CARTESIAN_POINT('',(87.0599996728755,45.5599996354697,380.));
#17518=CARTESIAN_POINT('',(86.0599996728755,44.5599996354697,380.));
#17519=CARTESIAN_POINT('Origin',(86.0599996824337,45.5599996259115,380.));
#17520=CARTESIAN_POINT('',(83.8599989099361,44.5599996354697,380.));
#17521=CARTESIAN_POINT('',(83.8599989099361,44.5599996354697,380.));
#17522=CARTESIAN_POINT('',(82.8599989099361,45.5599996354697,380.));
#17523=CARTESIAN_POINT('Origin',(83.8599989003778,45.5599996259115,380.));
#17524=CARTESIAN_POINT('',(82.8599989099361,47.7600003984092,380.));
#17525=CARTESIAN_POINT('',(82.859998909936,47.7600003984092,380.));
#17526=CARTESIAN_POINT('Origin',(83.8599989003778,47.7600004079674,380.));
#17527=CARTESIAN_POINT('Origin',(104.609999923724,22.4600011663401,0.));
#17528=CARTESIAN_POINT('',(95.6600000543452,29.0599999999999,0.));
#17529=CARTESIAN_POINT('',(96.5599999999999,29.5751481628425,0.));
#17530=CARTESIAN_POINT('',(95.6600000543452,29.0599999999999,0.));
#17531=CARTESIAN_POINT('',(92.3555338067866,29.0599999999999,0.));
#17532=CARTESIAN_POINT('',(92.3555338067866,29.0599999999999,0.));
#17533=CARTESIAN_POINT('',(88.3099996728755,25.0100007629401,0.));
#17534=CARTESIAN_POINT('',(88.3099996728755,25.0100007629401,0.));
#17535=CARTESIAN_POINT('',(88.3099996728755,22.4600011663401,0.));
#17536=CARTESIAN_POINT('',(88.3099996728755,22.4600011663401,0.));
#17537=CARTESIAN_POINT('',(88.5100000762757,22.2600007629398,0.));
#17538=CARTESIAN_POINT('Origin',(88.5100000762757,22.4600011663401,0.));
#17539=CARTESIAN_POINT('',(91.9099998030791,22.2600007629398,0.));
#17540=CARTESIAN_POINT('',(91.9099998030791,22.2600007629398,0.));
#17541=CARTESIAN_POINT('',(92.5099999999999,21.6600005660189,0.));
#17542=CARTESIAN_POINT('Origin',(91.9099998030791,21.6600005660189,0.));
#17543=CARTESIAN_POINT('',(92.5099999999999,20.7600003735979,0.));
#17544=CARTESIAN_POINT('',(92.5099999999999,20.7600003735979,0.));
#17545=CARTESIAN_POINT('',(92.309999626402,20.5599999999999,0.));
#17546=CARTESIAN_POINT('Origin',(92.309999626402,20.7600003735979,0.));
#17547=CARTESIAN_POINT('',(92.2099998557381,20.5599999999999,0.));
#17548=CARTESIAN_POINT('',(92.2099998557381,20.5599999999999,0.));
#17549=CARTESIAN_POINT('',(92.010000435814,20.3600005800758,0.));
#17550=CARTESIAN_POINT('Origin',(92.2099998557381,20.3600005800758,0.));
#17551=CARTESIAN_POINT('',(92.010000435814,20.2600003810484,0.));
#17552=CARTESIAN_POINT('',(92.010000435814,20.2600003810484,0.));
#17553=CARTESIAN_POINT('',(91.8100000547655,20.0599999999999,0.));
#17554=CARTESIAN_POINT('Origin',(91.8100000547655,20.2600003810484,0.));
#17555=CARTESIAN_POINT('',(83.5599996537578,20.0599999999999,0.));
#17556=CARTESIAN_POINT('',(83.5599996537578,20.0599999999999,0.));
#17557=CARTESIAN_POINT('',(81.5599999999999,22.0599996537577,0.));
#17558=CARTESIAN_POINT('Origin',(83.5599996537577,22.0599996537577,0.));
#17559=CARTESIAN_POINT('',(81.5599999999999,30.3100004787476,0.));
#17560=CARTESIAN_POINT('',(81.5599999999999,30.3100004787476,0.));
#17561=CARTESIAN_POINT('',(81.7600002841911,30.5100007629388,0.));
#17562=CARTESIAN_POINT('Origin',(81.7600002841911,30.3100004787476,0.));
#17563=CARTESIAN_POINT('',(81.8599993886842,30.5100007629388,0.));
#17564=CARTESIAN_POINT('',(81.8599993886842,30.5100007629388,0.));
#17565=CARTESIAN_POINT('',(82.0599996728754,30.71000104713,0.));
#17566=CARTESIAN_POINT('Origin',(81.8599993886842,30.71000104713,0.));
#17567=CARTESIAN_POINT('',(82.0599996728754,30.8100004787487,0.));
#17568=CARTESIAN_POINT('',(82.0599996728754,30.8100004787487,0.));
#17569=CARTESIAN_POINT('',(82.2599999570666,31.0100007629399,0.));
#17570=CARTESIAN_POINT('Origin',(82.2599999570666,30.8100004787487,0.));
#17571=CARTESIAN_POINT('',(83.1600000600806,31.0100007629399,0.));
#17572=CARTESIAN_POINT('',(83.1600000600806,31.0100007629399,0.));
#17573=CARTESIAN_POINT('',(83.7600004358154,30.4100003872052,0.));
#17574=CARTESIAN_POINT('Origin',(83.1600000600806,30.4100003872052,0.));
#17575=CARTESIAN_POINT('',(83.7600004358154,27.0100002841911,0.));
#17576=CARTESIAN_POINT('',(83.7600004358154,27.0100002841911,0.));
#17577=CARTESIAN_POINT('',(83.9600007200066,26.8099999999999,0.));
#17578=CARTESIAN_POINT('Origin',(83.9600007200066,27.0100002841911,0.));
#17579=CARTESIAN_POINT('',(86.510000435816,26.8099999999999,0.));
#17580=CARTESIAN_POINT('',(86.510000435816,26.8099999999999,0.));
#17581=CARTESIAN_POINT('',(90.5555345697271,30.8555341339111,0.));
#17582=CARTESIAN_POINT('',(90.5555345697271,30.8555341339111,0.));
#17583=CARTESIAN_POINT('',(90.5555345697271,34.1600003814696,0.));
#17584=CARTESIAN_POINT('',(90.5555345697271,34.1600003814696,0.));
#17585=CARTESIAN_POINT('',(91.0751478357183,35.0599999999999,0.));
#17586=CARTESIAN_POINT('',(91.0751478357183,35.0599999999999,0.));
#17587=CARTESIAN_POINT('',(90.5555345697271,35.9599996185302,0.));
#17588=CARTESIAN_POINT('',(90.5555345697271,35.9599996185302,0.));
#17589=CARTESIAN_POINT('',(90.5555345697271,39.2644658660888,0.));
#17590=CARTESIAN_POINT('',(90.5555345697271,39.2644658660888,0.));
#17591=CARTESIAN_POINT('',(86.510000435816,43.3099999999999,0.));
#17592=CARTESIAN_POINT('',(86.510000435816,43.3099999999999,0.));
#17593=CARTESIAN_POINT('',(83.9600007200066,43.3099999999999,0.));
#17594=CARTESIAN_POINT('',(83.9600007200066,43.3099999999999,0.));
#17595=CARTESIAN_POINT('',(83.7600004358154,43.1099997158087,0.));
#17596=CARTESIAN_POINT('Origin',(83.9600007200066,43.1099997158087,0.));
#17597=CARTESIAN_POINT('',(83.7600004358154,39.7099996127947,0.));
#17598=CARTESIAN_POINT('',(83.7600004358154,39.7099996127947,0.));
#17599=CARTESIAN_POINT('',(83.1600000600806,39.1099992370599,0.));
#17600=CARTESIAN_POINT('Origin',(83.1600000600806,39.7099996127947,0.));
#17601=CARTESIAN_POINT('',(82.2599999570666,39.1099992370599,0.));
#17602=CARTESIAN_POINT('',(82.2599999570666,39.1099992370599,0.));
#17603=CARTESIAN_POINT('',(82.0599996728754,39.3099995212511,0.));
#17604=CARTESIAN_POINT('Origin',(82.2599999570666,39.3099995212511,0.));
#17605=CARTESIAN_POINT('',(82.0599996728754,39.4099989528698,0.));
#17606=CARTESIAN_POINT('',(82.0599996728754,39.4099989528698,0.));
#17607=CARTESIAN_POINT('',(81.8599993886842,39.609999237061,0.));
#17608=CARTESIAN_POINT('Origin',(81.8599993886842,39.4099989528698,0.));
#17609=CARTESIAN_POINT('',(81.7600002841911,39.609999237061,0.));
#17610=CARTESIAN_POINT('',(81.7600002841911,39.609999237061,0.));
#17611=CARTESIAN_POINT('',(81.5599999999999,39.8099995212522,0.));
#17612=CARTESIAN_POINT('Origin',(81.7600002841911,39.8099995212522,0.));
#17613=CARTESIAN_POINT('',(81.5599999999999,48.0600003462421,0.));
#17614=CARTESIAN_POINT('',(81.5599999999999,48.0600003462421,0.));
#17615=CARTESIAN_POINT('',(83.5599996537577,50.0599999999999,0.));
#17616=CARTESIAN_POINT('Origin',(83.5599996537577,48.0600003462421,0.));
#17617=CARTESIAN_POINT('',(91.8100000547655,50.0599999999999,0.));
#17618=CARTESIAN_POINT('',(91.8100000547655,50.0599999999999,0.));
#17619=CARTESIAN_POINT('',(92.010000435814,49.8599996189514,0.));
#17620=CARTESIAN_POINT('Origin',(91.8100000547655,49.8599996189514,0.));
#17621=CARTESIAN_POINT('',(92.010000435814,49.759999419924,0.));
#17622=CARTESIAN_POINT('',(92.010000435814,49.759999419924,0.));
#17623=CARTESIAN_POINT('',(92.2099998557381,49.5599999999999,0.));
#17624=CARTESIAN_POINT('Origin',(92.2099998557381,49.759999419924,0.));
#17625=CARTESIAN_POINT('',(92.309999626402,49.5599999999999,0.));
#17626=CARTESIAN_POINT('',(92.309999626402,49.5599999999999,0.));
#17627=CARTESIAN_POINT('',(92.5099999999999,49.3599996264019,0.));
#17628=CARTESIAN_POINT('Origin',(92.309999626402,49.3599996264019,0.));
#17629=CARTESIAN_POINT('',(92.5099999999999,48.4599994339809,0.));
#17630=CARTESIAN_POINT('',(92.5099999999999,48.4599994339809,0.));
#17631=CARTESIAN_POINT('',(91.9099998030791,47.85999923706,0.));
#17632=CARTESIAN_POINT('Origin',(91.9099998030791,48.4599994339809,0.));
#17633=CARTESIAN_POINT('',(88.5100000762757,47.85999923706,0.));
#17634=CARTESIAN_POINT('',(88.5100000762757,47.85999923706,0.));
#17635=CARTESIAN_POINT('',(88.3099996728755,47.6599988336597,0.));
#17636=CARTESIAN_POINT('Origin',(88.5100000762757,47.6599988336597,0.));
#17637=CARTESIAN_POINT('',(88.3099996728755,45.1099992370597,0.));
#17638=CARTESIAN_POINT('',(88.3099996728755,45.1099992370597,0.));
#17639=CARTESIAN_POINT('',(92.3555338067866,41.0599999999999,0.));
#17640=CARTESIAN_POINT('',(92.3555338067866,41.0599999999999,0.));
#17641=CARTESIAN_POINT('',(95.6600000543452,41.0599999999999,0.));
#17642=CARTESIAN_POINT('',(95.6600000543452,41.0599999999999,0.));
#17643=CARTESIAN_POINT('',(96.5599999999999,40.5448518371574,0.));
#17644=CARTESIAN_POINT('',(96.5599999999999,40.5448518371574,0.));
#17645=CARTESIAN_POINT('',(97.4599999456547,41.0599999999999,0.));
#17646=CARTESIAN_POINT('',(97.4599999456547,41.0599999999999,0.));
#17647=CARTESIAN_POINT('',(100.764466193213,41.0599999999999,0.));
#17648=CARTESIAN_POINT('',(100.764466193213,41.0599999999999,0.));
#17649=CARTESIAN_POINT('',(104.810000327124,45.1099992370597,0.));
#17650=CARTESIAN_POINT('',(104.810000327124,45.1099992370597,0.));
#17651=CARTESIAN_POINT('',(104.810000327124,47.6599988336597,0.));
#17652=CARTESIAN_POINT('',(104.810000327124,47.6599988336597,0.));
#17653=CARTESIAN_POINT('',(104.609999923724,47.85999923706,0.));
#17654=CARTESIAN_POINT('Origin',(104.609999923724,47.6599988336597,0.));
#17655=CARTESIAN_POINT('',(101.210000196921,47.85999923706,0.));
#17656=CARTESIAN_POINT('',(101.210000196921,47.85999923706,0.));
#17657=CARTESIAN_POINT('',(100.61,48.4599994339809,0.));
#17658=CARTESIAN_POINT('Origin',(101.210000196921,48.4599994339809,0.));
#17659=CARTESIAN_POINT('',(100.61,49.3599996264019,0.));
#17660=CARTESIAN_POINT('',(100.61,49.3599996264019,0.));
#17661=CARTESIAN_POINT('',(100.810000373598,49.5599999999999,0.));
#17662=CARTESIAN_POINT('Origin',(100.810000373598,49.3599996264019,0.));
#17663=CARTESIAN_POINT('',(100.910000144262,49.5599999999999,0.));
#17664=CARTESIAN_POINT('',(100.910000144262,49.5599999999999,0.));
#17665=CARTESIAN_POINT('',(101.109999564186,49.759999419924,0.));
#17666=CARTESIAN_POINT('Origin',(100.910000144262,49.759999419924,0.));
#17667=CARTESIAN_POINT('',(101.109999564186,49.8599996189514,0.));
#17668=CARTESIAN_POINT('',(101.109999564186,49.8599996189514,0.));
#17669=CARTESIAN_POINT('',(101.309999945234,50.0599999999999,0.));
#17670=CARTESIAN_POINT('Origin',(101.309999945234,49.8599996189514,0.));
#17671=CARTESIAN_POINT('',(109.560000346242,50.0599999999999,0.));
#17672=CARTESIAN_POINT('',(109.560000346242,50.0599999999999,0.));
#17673=CARTESIAN_POINT('',(111.56,48.0600003462421,0.));
#17674=CARTESIAN_POINT('Origin',(109.560000346242,48.0600003462421,0.));
#17675=CARTESIAN_POINT('',(111.56,39.8099995212523,0.));
#17676=CARTESIAN_POINT('',(111.56,39.8099995212523,0.));
#17677=CARTESIAN_POINT('',(111.359999715809,39.609999237061,0.));
#17678=CARTESIAN_POINT('Origin',(111.359999715809,39.8099995212523,0.));
#17679=CARTESIAN_POINT('',(111.260000611316,39.609999237061,0.));
#17680=CARTESIAN_POINT('',(111.260000611316,39.609999237061,0.));
#17681=CARTESIAN_POINT('',(111.060000327124,39.4099989528698,0.));
#17682=CARTESIAN_POINT('Origin',(111.260000611316,39.4099989528698,0.));
#17683=CARTESIAN_POINT('',(111.060000327124,39.3099995212511,0.));
#17684=CARTESIAN_POINT('',(111.060000327124,39.3099995212511,0.));
#17685=CARTESIAN_POINT('',(110.860000042933,39.1099992370599,0.));
#17686=CARTESIAN_POINT('Origin',(110.860000042933,39.3099995212511,0.));
#17687=CARTESIAN_POINT('',(109.959999939919,39.1099992370599,0.));
#17688=CARTESIAN_POINT('',(109.959999939919,39.1099992370599,0.));
#17689=CARTESIAN_POINT('',(109.359999564184,39.7099996127947,0.));
#17690=CARTESIAN_POINT('Origin',(109.959999939919,39.7099996127947,0.));
#17691=CARTESIAN_POINT('',(109.359999564184,43.1099997158087,0.));
#17692=CARTESIAN_POINT('',(109.359999564184,43.1099997158087,0.));
#17693=CARTESIAN_POINT('',(109.159999279993,43.3099999999999,0.));
#17694=CARTESIAN_POINT('Origin',(109.159999279993,43.1099997158087,0.));
#17695=CARTESIAN_POINT('',(106.609999564184,43.3099999999999,0.));
#17696=CARTESIAN_POINT('',(106.609999564184,43.3099999999999,0.));
#17697=CARTESIAN_POINT('',(102.564465430273,39.2644658660888,0.));
#17698=CARTESIAN_POINT('',(102.564465430273,39.2644658660888,0.));
#17699=CARTESIAN_POINT('',(102.564465430273,35.9599996185302,0.));
#17700=CARTESIAN_POINT('',(102.564465430273,35.9599996185302,0.));
#17701=CARTESIAN_POINT('',(102.044852164282,35.0599999999999,0.));
#17702=CARTESIAN_POINT('',(102.044852164282,35.0599999999999,0.));
#17703=CARTESIAN_POINT('',(102.564465430273,34.1600003814696,0.));
#17704=CARTESIAN_POINT('',(102.564465430273,34.1600003814696,0.));
#17705=CARTESIAN_POINT('',(102.564465430273,30.8555341339111,0.));
#17706=CARTESIAN_POINT('',(102.564465430273,30.8555341339111,0.));
#17707=CARTESIAN_POINT('',(106.609999564184,26.8099999999999,0.));
#17708=CARTESIAN_POINT('',(106.609999564184,26.8099999999999,0.));
#17709=CARTESIAN_POINT('',(109.159999279993,26.8099999999999,0.));
#17710=CARTESIAN_POINT('',(109.159999279993,26.8099999999999,0.));
#17711=CARTESIAN_POINT('',(109.359999564184,27.0100002841911,0.));
#17712=CARTESIAN_POINT('Origin',(109.159999279993,27.0100002841911,0.));
#17713=CARTESIAN_POINT('',(109.359999564184,30.4100003872052,0.));
#17714=CARTESIAN_POINT('',(109.359999564184,30.4100003872052,0.));
#17715=CARTESIAN_POINT('',(109.959999939919,31.0100007629399,0.));
#17716=CARTESIAN_POINT('Origin',(109.959999939919,30.4100003872052,0.));
#17717=CARTESIAN_POINT('',(110.860000042933,31.0100007629399,0.));
#17718=CARTESIAN_POINT('',(110.860000042933,31.0100007629399,0.));
#17719=CARTESIAN_POINT('',(111.060000327124,30.8100004787487,0.));
#17720=CARTESIAN_POINT('Origin',(110.860000042933,30.8100004787487,0.));
#17721=CARTESIAN_POINT('',(111.060000327124,30.71000104713,0.));
#17722=CARTESIAN_POINT('',(111.060000327124,30.71000104713,0.));
#17723=CARTESIAN_POINT('',(111.260000611316,30.5100007629388,0.));
#17724=CARTESIAN_POINT('Origin',(111.260000611316,30.71000104713,0.));
#17725=CARTESIAN_POINT('',(111.359999715809,30.5100007629388,0.));
#17726=CARTESIAN_POINT('',(111.359999715809,30.5100007629388,0.));
#17727=CARTESIAN_POINT('',(111.56,30.3100004787476,0.));
#17728=CARTESIAN_POINT('Origin',(111.359999715809,30.3100004787476,0.));
#17729=CARTESIAN_POINT('',(111.56,22.0599996537577,0.));
#17730=CARTESIAN_POINT('',(111.56,22.0599996537577,0.));
#17731=CARTESIAN_POINT('',(109.560000346242,20.0599999999999,0.));
#17732=CARTESIAN_POINT('Origin',(109.560000346242,22.0599996537577,0.));
#17733=CARTESIAN_POINT('',(101.309999945234,20.0599999999999,0.));
#17734=CARTESIAN_POINT('',(101.309999945234,20.0599999999999,0.));
#17735=CARTESIAN_POINT('',(101.109999564186,20.2600003810484,0.));
#17736=CARTESIAN_POINT('Origin',(101.309999945234,20.2600003810484,0.));
#17737=CARTESIAN_POINT('',(101.109999564186,20.3600005800758,0.));
#17738=CARTESIAN_POINT('',(101.109999564186,20.3600005800758,0.));
#17739=CARTESIAN_POINT('',(100.910000144262,20.5599999999999,0.));
#17740=CARTESIAN_POINT('Origin',(100.910000144262,20.3600005800758,0.));
#17741=CARTESIAN_POINT('',(100.810000373598,20.5599999999999,0.));
#17742=CARTESIAN_POINT('',(100.810000373598,20.5599999999999,0.));
#17743=CARTESIAN_POINT('',(100.61,20.7600003735979,0.));
#17744=CARTESIAN_POINT('Origin',(100.810000373598,20.7600003735979,0.));
#17745=CARTESIAN_POINT('',(100.61,21.6600005660189,0.));
#17746=CARTESIAN_POINT('',(100.61,21.6600005660189,0.));
#17747=CARTESIAN_POINT('',(101.210000196921,22.2600007629398,0.));
#17748=CARTESIAN_POINT('Origin',(101.210000196921,21.6600005660189,0.));
#17749=CARTESIAN_POINT('',(104.609999923724,22.2600007629398,0.));
#17750=CARTESIAN_POINT('',(104.609999923724,22.2600007629398,0.));
#17751=CARTESIAN_POINT('',(104.810000327124,22.4600011663401,0.));
#17752=CARTESIAN_POINT('Origin',(104.609999923724,22.4600011663401,0.));
#17753=CARTESIAN_POINT('',(104.810000327124,25.0100007629401,0.));
#17754=CARTESIAN_POINT('',(104.810000327124,25.0100007629401,0.));
#17755=CARTESIAN_POINT('',(100.764466193213,29.0599999999999,0.));
#17756=CARTESIAN_POINT('',(100.764466193213,29.0599999999999,0.));
#17757=CARTESIAN_POINT('',(97.4599999456547,29.0599999999999,0.));
#17758=CARTESIAN_POINT('',(97.4599999456547,29.0599999999999,0.));
#17759=CARTESIAN_POINT('',(96.5599999999999,29.5751481628425,0.));
#17760=CARTESIAN_POINT('',(110.260001090064,47.7600003984092,0.));
#17761=CARTESIAN_POINT('',(109.260001090064,48.7600003984092,0.));
#17762=CARTESIAN_POINT('Origin',(109.260001099622,47.7600004079674,0.));
#17763=CARTESIAN_POINT('',(107.060000327124,48.7600003984092,0.));
#17764=CARTESIAN_POINT('',(109.260001090064,48.7600003984092,0.));
#17765=CARTESIAN_POINT('',(106.060000327124,47.7600003984092,0.));
#17766=CARTESIAN_POINT('Origin',(107.060000317566,47.7600004079674,0.));
#17767=CARTESIAN_POINT('',(106.060000327124,45.5599996354697,0.));
#17768=CARTESIAN_POINT('',(106.060000327124,47.7600003984092,0.));
#17769=CARTESIAN_POINT('',(107.060000327124,44.5599996354697,0.));
#17770=CARTESIAN_POINT('Origin',(107.060000317566,45.5599996259115,0.));
#17771=CARTESIAN_POINT('',(109.260001090064,44.5599996354697,0.));
#17772=CARTESIAN_POINT('',(107.060000327124,44.5599996354697,0.));
#17773=CARTESIAN_POINT('',(110.260001090064,45.5599996354697,0.));
#17774=CARTESIAN_POINT('Origin',(109.260001099622,45.5599996259115,0.));
#17775=CARTESIAN_POINT('',(110.260001090064,45.5599996354697,0.));
#17776=CARTESIAN_POINT('',(82.8599989099361,22.3599996015906,0.));
#17777=CARTESIAN_POINT('',(83.859998909936,21.3599996015906,0.));
#17778=CARTESIAN_POINT('Origin',(83.8599989003778,22.3599995920324,0.));
#17779=CARTESIAN_POINT('',(86.0599996728755,21.3599996015906,0.));
#17780=CARTESIAN_POINT('',(83.859998909936,21.3599996015906,0.));
#17781=CARTESIAN_POINT('',(87.0599996728755,22.3599996015906,0.));
#17782=CARTESIAN_POINT('Origin',(86.0599996824337,22.3599995920324,0.));
#17783=CARTESIAN_POINT('',(87.0599996728755,24.5600003645301,0.));
#17784=CARTESIAN_POINT('',(87.0599996728755,22.3599996015906,0.));
#17785=CARTESIAN_POINT('',(86.0599996728755,25.5600003645301,0.));
#17786=CARTESIAN_POINT('Origin',(86.0599996824337,24.5600003740883,0.));
#17787=CARTESIAN_POINT('',(83.859998909936,25.5600003645301,0.));
#17788=CARTESIAN_POINT('',(86.0599996728755,25.5600003645301,0.));
#17789=CARTESIAN_POINT('',(82.8599989099361,24.5600003645301,0.));
#17790=CARTESIAN_POINT('Origin',(83.8599989003778,24.5600003740883,0.));
#17791=CARTESIAN_POINT('',(82.859998909936,24.5600003645301,0.));
#17792=CARTESIAN_POINT('',(87.0599996728755,47.7600003984092,0.));
#17793=CARTESIAN_POINT('',(86.0599996728755,48.7600003984092,0.));
#17794=CARTESIAN_POINT('Origin',(86.0599996824337,47.7600004079674,0.));
#17795=CARTESIAN_POINT('',(83.859998909936,48.7600003984092,0.));
#17796=CARTESIAN_POINT('',(86.0599996728755,48.7600003984092,0.));
#17797=CARTESIAN_POINT('',(82.8599989099361,47.7600003984092,0.));
#17798=CARTESIAN_POINT('Origin',(83.8599989003778,47.7600004079674,0.));
#17799=CARTESIAN_POINT('',(82.8599989099361,45.5599996354697,0.));
#17800=CARTESIAN_POINT('',(82.859998909936,47.7600003984092,0.));
#17801=CARTESIAN_POINT('',(83.8599989099361,44.5599996354697,0.));
#17802=CARTESIAN_POINT('Origin',(83.8599989003778,45.5599996259115,0.));
#17803=CARTESIAN_POINT('',(86.0599996728755,44.5599996354697,0.));
#17804=CARTESIAN_POINT('',(83.8599989099361,44.5599996354697,0.));
#17805=CARTESIAN_POINT('',(87.0599996728755,45.5599996354697,0.));
#17806=CARTESIAN_POINT('Origin',(86.0599996824337,45.5599996259115,0.));
#17807=CARTESIAN_POINT('',(87.0599996728755,45.5599996354697,0.));
#17808=CARTESIAN_POINT('',(109.260001090064,21.3599996015906,0.));
#17809=CARTESIAN_POINT('',(110.260001090064,22.3599996015906,0.));
#17810=CARTESIAN_POINT('Origin',(109.260001099622,22.3599995920324,0.));
#17811=CARTESIAN_POINT('',(110.260001090064,24.5600003645301,0.));
#17812=CARTESIAN_POINT('',(110.260001090064,22.3599996015906,0.));
#17813=CARTESIAN_POINT('',(109.260001090064,25.5600003645301,0.));
#17814=CARTESIAN_POINT('Origin',(109.260001099622,24.5600003740883,0.));
#17815=CARTESIAN_POINT('',(107.060000327124,25.5600003645301,0.));
#17816=CARTESIAN_POINT('',(109.260001090064,25.5600003645301,0.));
#17817=CARTESIAN_POINT('',(106.060000327124,24.5600003645301,0.));
#17818=CARTESIAN_POINT('Origin',(107.060000317566,24.5600003740883,0.));
#17819=CARTESIAN_POINT('',(106.060000327124,22.3599996015906,0.));
#17820=CARTESIAN_POINT('',(106.060000327124,24.5600003645301,0.));
#17821=CARTESIAN_POINT('',(107.060000327124,21.3599996015906,0.));
#17822=CARTESIAN_POINT('Origin',(107.060000317566,22.3599995920324,0.));
#17823=CARTESIAN_POINT('',(107.060000327124,21.3599996015906,0.));
#17824=CARTESIAN_POINT('',(98.1601295238092,38.3405617669895,0.));
#17825=CARTESIAN_POINT('',(94.9598704761907,38.3405617669895,0.));
#17826=CARTESIAN_POINT('Origin',(96.5599999999999,35.0599999999999,0.));
#17827=CARTESIAN_POINT('',(93.4240705880017,39.5784009033024,0.));
#17828=CARTESIAN_POINT('',(94.9598704761907,38.3405617669895,0.));
#17829=CARTESIAN_POINT('',(92.0546631075751,38.2146694732975,0.));
#17830=CARTESIAN_POINT('Origin',(96.5599999999999,35.0599999999999,0.));
#17831=CARTESIAN_POINT('',(92.0546631075751,38.2146694732975,0.));
#17832=CARTESIAN_POINT('',(92.0546631075751,31.9053305267024,0.));
#17833=CARTESIAN_POINT('',(93.279438268468,33.4598704034959,0.));
#17834=CARTESIAN_POINT('',(93.4240705880018,30.5415990966974,0.));
#17835=CARTESIAN_POINT('Origin',(96.5599999999999,35.0599999999999,0.));
#17836=CARTESIAN_POINT('',(94.9598704761907,31.7794382330103,0.));
#17837=CARTESIAN_POINT('',(93.4240705880018,30.5415990966974,0.));
#17838=CARTESIAN_POINT('',(98.1601295238092,31.7794382330103,0.));
#17839=CARTESIAN_POINT('Origin',(96.5599999999999,35.0599999999999,0.));
#17840=CARTESIAN_POINT('',(99.6959294119981,30.5415990966974,0.));
#17841=CARTESIAN_POINT('',(98.1601295238092,31.7794382330103,0.));
#17842=CARTESIAN_POINT('',(101.065336892425,31.9053305267024,0.));
#17843=CARTESIAN_POINT('Origin',(96.5599999999999,35.0599999999999,0.));
#17844=CARTESIAN_POINT('',(99.8405617315319,33.459870403496,0.));
#17845=CARTESIAN_POINT('',(101.065336892425,31.9053305267024,0.));
#17846=CARTESIAN_POINT('',(99.8405617315319,36.6601295965039,0.));
#17847=CARTESIAN_POINT('Origin',(96.5599999999999,35.0599999999999,0.));
#17848=CARTESIAN_POINT('',(101.065336892425,38.2146694732975,0.));
#17849=CARTESIAN_POINT('',(99.8405617315319,36.6601295965039,0.));
#17850=CARTESIAN_POINT('',(99.6959294119981,39.5784009033024,0.));
#17851=CARTESIAN_POINT('Origin',(96.5599999999999,35.0599999999999,0.));
#17852=CARTESIAN_POINT('',(99.6959294119981,39.5784009033024,0.));
#17853=CARTESIAN_POINT('Origin',(95.6600000543452,29.0599999999999,380.));
#17854=CARTESIAN_POINT('',(96.5599999999999,29.5751481628425,380.));
#17855=CARTESIAN_POINT('',(95.6600000543452,29.0599999999999,380.));
#17856=CARTESIAN_POINT('Origin',(96.5599999999999,29.5751481628425,380.));
#17857=CARTESIAN_POINT('',(97.4599999456547,29.0599999999999,380.));
#17858=CARTESIAN_POINT('Origin',(97.4599999456547,29.0599999999999,380.));
#17859=CARTESIAN_POINT('',(100.764466193213,29.0599999999999,380.));
#17860=CARTESIAN_POINT('Origin',(100.764466193213,29.0599999999999,380.));
#17861=CARTESIAN_POINT('',(104.810000327124,25.0100007629401,380.));
#17862=CARTESIAN_POINT('Origin',(104.810000327124,25.0100007629401,380.));
#17863=CARTESIAN_POINT('',(104.810000327124,22.4600011663401,380.));
#17864=CARTESIAN_POINT('Origin',(104.609999923724,22.4600011663401,380.));
#17865=CARTESIAN_POINT('',(104.609999923724,22.2600007629398,380.));
#17866=CARTESIAN_POINT('Origin',(104.609999923724,22.2600007629398,380.));
#17867=CARTESIAN_POINT('',(101.210000196921,22.2600007629398,380.));
#17868=CARTESIAN_POINT('Origin',(101.210000196921,21.6600005660189,380.));
#17869=CARTESIAN_POINT('',(100.61,21.6600005660189,380.));
#17870=CARTESIAN_POINT('Origin',(100.61,21.6600005660189,380.));
#17871=CARTESIAN_POINT('',(100.61,20.7600003735979,380.));
#17872=CARTESIAN_POINT('Origin',(100.810000373598,20.7600003735979,380.));
#17873=CARTESIAN_POINT('',(100.810000373598,20.5599999999999,380.));
#17874=CARTESIAN_POINT('Origin',(100.810000373598,20.5599999999999,380.));
#17875=CARTESIAN_POINT('',(100.910000144262,20.5599999999999,380.));
#17876=CARTESIAN_POINT('Origin',(100.910000144262,20.3600005800758,380.));
#17877=CARTESIAN_POINT('',(101.109999564186,20.3600005800758,380.));
#17878=CARTESIAN_POINT('Origin',(101.109999564186,20.3600005800758,380.));
#17879=CARTESIAN_POINT('',(101.109999564186,20.2600003810484,380.));
#17880=CARTESIAN_POINT('Origin',(101.309999945234,20.2600003810484,380.));
#17881=CARTESIAN_POINT('',(101.309999945234,20.0599999999999,380.));
#17882=CARTESIAN_POINT('Origin',(101.309999945234,20.0599999999999,380.));
#17883=CARTESIAN_POINT('',(109.560000346242,20.0599999999999,380.));
#17884=CARTESIAN_POINT('Origin',(109.560000346242,22.0599996537577,380.));
#17885=CARTESIAN_POINT('',(111.56,22.0599996537577,380.));
#17886=CARTESIAN_POINT('Origin',(111.56,22.0599996537577,380.));
#17887=CARTESIAN_POINT('',(111.56,30.3100004787476,380.));
#17888=CARTESIAN_POINT('Origin',(111.359999715809,30.3100004787476,380.));
#17889=CARTESIAN_POINT('',(111.359999715809,30.5100007629388,380.));
#17890=CARTESIAN_POINT('Origin',(111.359999715809,30.5100007629388,380.));
#17891=CARTESIAN_POINT('',(111.260000611316,30.5100007629388,380.));
#17892=CARTESIAN_POINT('Origin',(111.260000611316,30.71000104713,380.));
#17893=CARTESIAN_POINT('',(111.060000327124,30.71000104713,380.));
#17894=CARTESIAN_POINT('Origin',(111.060000327124,30.71000104713,380.));
#17895=CARTESIAN_POINT('',(111.060000327124,30.8100004787487,380.));
#17896=CARTESIAN_POINT('Origin',(110.860000042933,30.8100004787487,380.));
#17897=CARTESIAN_POINT('',(110.860000042933,31.0100007629399,380.));
#17898=CARTESIAN_POINT('Origin',(110.860000042933,31.0100007629399,380.));
#17899=CARTESIAN_POINT('',(109.959999939919,31.0100007629399,380.));
#17900=CARTESIAN_POINT('Origin',(109.959999939919,30.4100003872052,380.));
#17901=CARTESIAN_POINT('',(109.359999564184,30.4100003872052,380.));
#17902=CARTESIAN_POINT('Origin',(109.359999564184,30.4100003872052,380.));
#17903=CARTESIAN_POINT('',(109.359999564184,27.0100002841911,380.));
#17904=CARTESIAN_POINT('Origin',(109.159999279993,27.0100002841911,380.));
#17905=CARTESIAN_POINT('',(109.159999279993,26.8099999999999,380.));
#17906=CARTESIAN_POINT('Origin',(109.159999279993,26.8099999999999,380.));
#17907=CARTESIAN_POINT('',(106.609999564184,26.8099999999999,380.));
#17908=CARTESIAN_POINT('Origin',(106.609999564184,26.8099999999999,380.));
#17909=CARTESIAN_POINT('',(102.564465430273,30.8555341339111,380.));
#17910=CARTESIAN_POINT('Origin',(102.564465430273,30.8555341339111,380.));
#17911=CARTESIAN_POINT('',(102.564465430273,34.1600003814696,380.));
#17912=CARTESIAN_POINT('Origin',(102.564465430273,34.1600003814696,380.));
#17913=CARTESIAN_POINT('',(102.044852164282,35.0599999999999,380.));
#17914=CARTESIAN_POINT('Origin',(102.044852164282,35.0599999999999,380.));
#17915=CARTESIAN_POINT('',(102.564465430273,35.9599996185302,380.));
#17916=CARTESIAN_POINT('Origin',(102.564465430273,35.9599996185302,380.));
#17917=CARTESIAN_POINT('',(102.564465430273,39.2644658660888,380.));
#17918=CARTESIAN_POINT('Origin',(102.564465430273,39.2644658660888,380.));
#17919=CARTESIAN_POINT('',(106.609999564184,43.3099999999999,380.));
#17920=CARTESIAN_POINT('Origin',(106.609999564184,43.3099999999999,380.));
#17921=CARTESIAN_POINT('',(109.159999279993,43.3099999999999,380.));
#17922=CARTESIAN_POINT('Origin',(109.159999279993,43.1099997158087,380.));
#17923=CARTESIAN_POINT('',(109.359999564184,43.1099997158087,380.));
#17924=CARTESIAN_POINT('Origin',(109.359999564184,43.1099997158087,380.));
#17925=CARTESIAN_POINT('',(109.359999564184,39.7099996127947,380.));
#17926=CARTESIAN_POINT('Origin',(109.959999939919,39.7099996127947,380.));
#17927=CARTESIAN_POINT('',(109.959999939919,39.1099992370599,380.));
#17928=CARTESIAN_POINT('Origin',(109.959999939919,39.1099992370599,380.));
#17929=CARTESIAN_POINT('',(110.860000042933,39.1099992370599,380.));
#17930=CARTESIAN_POINT('Origin',(110.860000042933,39.3099995212511,380.));
#17931=CARTESIAN_POINT('',(111.060000327124,39.3099995212511,380.));
#17932=CARTESIAN_POINT('Origin',(111.060000327124,39.3099995212511,380.));
#17933=CARTESIAN_POINT('',(111.060000327124,39.4099989528698,380.));
#17934=CARTESIAN_POINT('Origin',(111.260000611316,39.4099989528698,380.));
#17935=CARTESIAN_POINT('',(111.260000611316,39.609999237061,380.));
#17936=CARTESIAN_POINT('Origin',(111.260000611316,39.609999237061,380.));
#17937=CARTESIAN_POINT('',(111.359999715809,39.609999237061,380.));
#17938=CARTESIAN_POINT('Origin',(111.359999715809,39.8099995212523,380.));
#17939=CARTESIAN_POINT('',(111.56,39.8099995212523,380.));
#17940=CARTESIAN_POINT('Origin',(111.56,39.8099995212523,380.));
#17941=CARTESIAN_POINT('',(111.56,48.0600003462421,380.));
#17942=CARTESIAN_POINT('Origin',(109.560000346242,48.0600003462421,380.));
#17943=CARTESIAN_POINT('',(109.560000346242,50.0599999999999,380.));
#17944=CARTESIAN_POINT('Origin',(109.560000346242,50.0599999999999,380.));
#17945=CARTESIAN_POINT('',(101.309999945234,50.0599999999999,380.));
#17946=CARTESIAN_POINT('Origin',(101.309999945234,49.8599996189514,380.));
#17947=CARTESIAN_POINT('',(101.109999564186,49.8599996189514,380.));
#17948=CARTESIAN_POINT('Origin',(101.109999564186,49.8599996189514,380.));
#17949=CARTESIAN_POINT('',(101.109999564186,49.759999419924,380.));
#17950=CARTESIAN_POINT('Origin',(100.910000144262,49.759999419924,380.));
#17951=CARTESIAN_POINT('',(100.910000144262,49.5599999999999,380.));
#17952=CARTESIAN_POINT('Origin',(100.910000144262,49.5599999999999,380.));
#17953=CARTESIAN_POINT('',(100.810000373598,49.5599999999999,380.));
#17954=CARTESIAN_POINT('Origin',(100.810000373598,49.3599996264019,380.));
#17955=CARTESIAN_POINT('',(100.61,49.3599996264019,380.));
#17956=CARTESIAN_POINT('Origin',(100.61,49.3599996264019,380.));
#17957=CARTESIAN_POINT('',(100.61,48.4599994339809,380.));
#17958=CARTESIAN_POINT('Origin',(101.210000196921,48.4599994339809,380.));
#17959=CARTESIAN_POINT('',(101.210000196921,47.85999923706,380.));
#17960=CARTESIAN_POINT('Origin',(101.210000196921,47.85999923706,380.));
#17961=CARTESIAN_POINT('',(104.609999923724,47.85999923706,380.));
#17962=CARTESIAN_POINT('Origin',(104.609999923724,47.6599988336597,380.));
#17963=CARTESIAN_POINT('',(104.810000327124,47.6599988336597,380.));
#17964=CARTESIAN_POINT('Origin',(104.810000327124,47.6599988336597,380.));
#17965=CARTESIAN_POINT('',(104.810000327124,45.1099992370597,380.));
#17966=CARTESIAN_POINT('Origin',(104.810000327124,45.1099992370597,380.));
#17967=CARTESIAN_POINT('',(100.764466193213,41.0599999999999,380.));
#17968=CARTESIAN_POINT('Origin',(100.764466193213,41.0599999999999,380.));
#17969=CARTESIAN_POINT('',(97.4599999456547,41.0599999999999,380.));
#17970=CARTESIAN_POINT('Origin',(97.4599999456547,41.0599999999999,380.));
#17971=CARTESIAN_POINT('',(96.5599999999999,40.5448518371574,380.));
#17972=CARTESIAN_POINT('Origin',(96.5599999999999,40.5448518371574,380.));
#17973=CARTESIAN_POINT('',(95.6600000543452,41.0599999999999,380.));
#17974=CARTESIAN_POINT('Origin',(95.6600000543452,41.0599999999999,380.));
#17975=CARTESIAN_POINT('',(92.3555338067866,41.0599999999999,380.));
#17976=CARTESIAN_POINT('Origin',(92.3555338067866,41.0599999999999,380.));
#17977=CARTESIAN_POINT('',(88.3099996728755,45.1099992370597,380.));
#17978=CARTESIAN_POINT('Origin',(88.3099996728755,45.1099992370597,380.));
#17979=CARTESIAN_POINT('',(88.3099996728755,47.6599988336597,380.));
#17980=CARTESIAN_POINT('Origin',(88.5100000762757,47.6599988336597,380.));
#17981=CARTESIAN_POINT('',(88.5100000762757,47.85999923706,380.));
#17982=CARTESIAN_POINT('Origin',(88.5100000762757,47.85999923706,380.));
#17983=CARTESIAN_POINT('',(91.9099998030791,47.85999923706,380.));
#17984=CARTESIAN_POINT('Origin',(91.9099998030791,48.4599994339809,380.));
#17985=CARTESIAN_POINT('',(92.5099999999999,48.4599994339809,380.));
#17986=CARTESIAN_POINT('Origin',(92.5099999999999,48.4599994339809,380.));
#17987=CARTESIAN_POINT('',(92.5099999999999,49.3599996264019,380.));
#17988=CARTESIAN_POINT('Origin',(92.309999626402,49.3599996264019,380.));
#17989=CARTESIAN_POINT('',(92.309999626402,49.5599999999999,380.));
#17990=CARTESIAN_POINT('Origin',(92.309999626402,49.5599999999999,380.));
#17991=CARTESIAN_POINT('',(92.2099998557381,49.5599999999999,380.));
#17992=CARTESIAN_POINT('Origin',(92.2099998557381,49.759999419924,380.));
#17993=CARTESIAN_POINT('',(92.010000435814,49.759999419924,380.));
#17994=CARTESIAN_POINT('Origin',(92.010000435814,49.759999419924,380.));
#17995=CARTESIAN_POINT('',(92.010000435814,49.8599996189514,380.));
#17996=CARTESIAN_POINT('Origin',(91.8100000547655,49.8599996189514,380.));
#17997=CARTESIAN_POINT('',(91.8100000547655,50.0599999999999,380.));
#17998=CARTESIAN_POINT('Origin',(91.8100000547655,50.0599999999999,380.));
#17999=CARTESIAN_POINT('',(83.5599996537577,50.0599999999999,380.));
#18000=CARTESIAN_POINT('Origin',(83.5599996537577,48.0600003462421,380.));
#18001=CARTESIAN_POINT('',(81.5599999999999,48.0600003462421,380.));
#18002=CARTESIAN_POINT('Origin',(81.5599999999999,48.0600003462421,380.));
#18003=CARTESIAN_POINT('',(81.5599999999999,39.8099995212522,380.));
#18004=CARTESIAN_POINT('Origin',(81.7600002841911,39.8099995212522,380.));
#18005=CARTESIAN_POINT('',(81.7600002841911,39.609999237061,380.));
#18006=CARTESIAN_POINT('Origin',(81.7600002841911,39.609999237061,380.));
#18007=CARTESIAN_POINT('',(81.8599993886842,39.609999237061,380.));
#18008=CARTESIAN_POINT('Origin',(81.8599993886842,39.4099989528698,380.));
#18009=CARTESIAN_POINT('',(82.0599996728754,39.4099989528698,380.));
#18010=CARTESIAN_POINT('Origin',(82.0599996728754,39.4099989528698,380.));
#18011=CARTESIAN_POINT('',(82.0599996728754,39.3099995212511,380.));
#18012=CARTESIAN_POINT('Origin',(82.2599999570666,39.3099995212511,380.));
#18013=CARTESIAN_POINT('',(82.2599999570666,39.1099992370599,380.));
#18014=CARTESIAN_POINT('Origin',(82.2599999570666,39.1099992370599,380.));
#18015=CARTESIAN_POINT('',(83.1600000600806,39.1099992370599,380.));
#18016=CARTESIAN_POINT('Origin',(83.1600000600806,39.7099996127947,380.));
#18017=CARTESIAN_POINT('',(83.7600004358154,39.7099996127947,380.));
#18018=CARTESIAN_POINT('Origin',(83.7600004358154,39.7099996127947,380.));
#18019=CARTESIAN_POINT('',(83.7600004358154,43.1099997158087,380.));
#18020=CARTESIAN_POINT('Origin',(83.9600007200066,43.1099997158087,380.));
#18021=CARTESIAN_POINT('',(83.9600007200066,43.3099999999999,380.));
#18022=CARTESIAN_POINT('Origin',(83.9600007200066,43.3099999999999,380.));
#18023=CARTESIAN_POINT('',(86.510000435816,43.3099999999999,380.));
#18024=CARTESIAN_POINT('Origin',(86.510000435816,43.3099999999999,380.));
#18025=CARTESIAN_POINT('',(90.5555345697271,39.2644658660888,380.));
#18026=CARTESIAN_POINT('Origin',(90.5555345697271,39.2644658660888,380.));
#18027=CARTESIAN_POINT('',(90.5555345697271,35.9599996185302,380.));
#18028=CARTESIAN_POINT('Origin',(90.5555345697271,35.9599996185302,380.));
#18029=CARTESIAN_POINT('',(91.0751478357183,35.0599999999999,380.));
#18030=CARTESIAN_POINT('Origin',(91.0751478357183,35.0599999999999,380.));
#18031=CARTESIAN_POINT('',(90.5555345697271,34.1600003814696,380.));
#18032=CARTESIAN_POINT('Origin',(90.5555345697271,34.1600003814696,380.));
#18033=CARTESIAN_POINT('',(90.5555345697271,30.8555341339111,380.));
#18034=CARTESIAN_POINT('Origin',(90.5555345697271,30.8555341339111,380.));
#18035=CARTESIAN_POINT('',(86.510000435816,26.8099999999999,380.));
#18036=CARTESIAN_POINT('Origin',(86.510000435816,26.8099999999999,380.));
#18037=CARTESIAN_POINT('',(83.9600007200066,26.8099999999999,380.));
#18038=CARTESIAN_POINT('Origin',(83.9600007200066,27.0100002841911,380.));
#18039=CARTESIAN_POINT('',(83.7600004358154,27.0100002841911,380.));
#18040=CARTESIAN_POINT('Origin',(83.7600004358154,27.0100002841911,380.));
#18041=CARTESIAN_POINT('',(83.7600004358154,30.4100003872052,380.));
#18042=CARTESIAN_POINT('Origin',(83.1600000600806,30.4100003872052,380.));
#18043=CARTESIAN_POINT('',(83.1600000600806,31.0100007629399,380.));
#18044=CARTESIAN_POINT('Origin',(83.1600000600806,31.0100007629399,380.));
#18045=CARTESIAN_POINT('',(82.2599999570666,31.0100007629399,380.));
#18046=CARTESIAN_POINT('Origin',(82.2599999570666,30.8100004787487,380.));
#18047=CARTESIAN_POINT('',(82.0599996728754,30.8100004787487,380.));
#18048=CARTESIAN_POINT('Origin',(82.0599996728754,30.8100004787487,380.));
#18049=CARTESIAN_POINT('',(82.0599996728754,30.71000104713,380.));
#18050=CARTESIAN_POINT('Origin',(81.8599993886842,30.71000104713,380.));
#18051=CARTESIAN_POINT('',(81.8599993886842,30.5100007629388,380.));
#18052=CARTESIAN_POINT('Origin',(81.8599993886842,30.5100007629388,380.));
#18053=CARTESIAN_POINT('',(81.7600002841911,30.5100007629388,380.));
#18054=CARTESIAN_POINT('Origin',(81.7600002841911,30.3100004787476,380.));
#18055=CARTESIAN_POINT('',(81.5599999999999,30.3100004787476,380.));
#18056=CARTESIAN_POINT('Origin',(81.5599999999999,30.3100004787476,380.));
#18057=CARTESIAN_POINT('',(81.5599999999999,22.0599996537577,380.));
#18058=CARTESIAN_POINT('Origin',(83.5599996537577,22.0599996537577,380.));
#18059=CARTESIAN_POINT('',(83.5599996537578,20.0599999999999,380.));
#18060=CARTESIAN_POINT('Origin',(83.5599996537578,20.0599999999999,380.));
#18061=CARTESIAN_POINT('',(91.8100000547655,20.0599999999999,380.));
#18062=CARTESIAN_POINT('Origin',(91.8100000547655,20.2600003810484,380.));
#18063=CARTESIAN_POINT('',(92.010000435814,20.2600003810484,380.));
#18064=CARTESIAN_POINT('Origin',(92.010000435814,20.2600003810484,380.));
#18065=CARTESIAN_POINT('',(92.010000435814,20.3600005800758,380.));
#18066=CARTESIAN_POINT('Origin',(92.2099998557381,20.3600005800758,380.));
#18067=CARTESIAN_POINT('',(92.2099998557381,20.5599999999999,380.));
#18068=CARTESIAN_POINT('Origin',(92.2099998557381,20.5599999999999,380.));
#18069=CARTESIAN_POINT('',(92.309999626402,20.5599999999999,380.));
#18070=CARTESIAN_POINT('Origin',(92.309999626402,20.7600003735979,380.));
#18071=CARTESIAN_POINT('',(92.5099999999999,20.7600003735979,380.));
#18072=CARTESIAN_POINT('Origin',(92.5099999999999,20.7600003735979,380.));
#18073=CARTESIAN_POINT('',(92.5099999999999,21.6600005660189,380.));
#18074=CARTESIAN_POINT('Origin',(91.9099998030791,21.6600005660189,380.));
#18075=CARTESIAN_POINT('',(91.9099998030791,22.2600007629398,380.));
#18076=CARTESIAN_POINT('Origin',(91.9099998030791,22.2600007629398,380.));
#18077=CARTESIAN_POINT('',(88.5100000762757,22.2600007629398,380.));
#18078=CARTESIAN_POINT('Origin',(88.5100000762757,22.4600011663401,380.));
#18079=CARTESIAN_POINT('',(88.3099996728755,22.4600011663401,380.));
#18080=CARTESIAN_POINT('Origin',(88.3099996728755,22.4600011663401,380.));
#18081=CARTESIAN_POINT('',(88.3099996728755,25.0100007629401,380.));
#18082=CARTESIAN_POINT('Origin',(88.3099996728755,25.0100007629401,380.));
#18083=CARTESIAN_POINT('',(92.3555338067866,29.0599999999999,380.));
#18084=CARTESIAN_POINT('Origin',(92.3555338067866,29.0599999999999,380.));
#18085=CARTESIAN_POINT('Origin',(109.260001099622,47.7600004079674,380.));
#18086=CARTESIAN_POINT('',(110.260001090064,47.7600003984092,380.));
#18087=CARTESIAN_POINT('',(109.260001090064,48.7600003984092,380.));
#18088=CARTESIAN_POINT('Origin',(109.260001090064,48.7600003984092,380.));
#18089=CARTESIAN_POINT('',(107.060000327124,48.7600003984092,380.));
#18090=CARTESIAN_POINT('Origin',(107.060000317566,47.7600004079674,380.));
#18091=CARTESIAN_POINT('',(106.060000327124,47.7600003984092,380.));
#18092=CARTESIAN_POINT('Origin',(106.060000327124,47.7600003984092,380.));
#18093=CARTESIAN_POINT('',(106.060000327124,45.5599996354697,380.));
#18094=CARTESIAN_POINT('Origin',(107.060000317566,45.5599996259115,380.));
#18095=CARTESIAN_POINT('',(107.060000327124,44.5599996354697,380.));
#18096=CARTESIAN_POINT('Origin',(107.060000327124,44.5599996354697,380.));
#18097=CARTESIAN_POINT('',(109.260001090064,44.5599996354697,380.));
#18098=CARTESIAN_POINT('Origin',(109.260001099622,45.5599996259115,380.));
#18099=CARTESIAN_POINT('',(110.260001090064,45.5599996354697,380.));
#18100=CARTESIAN_POINT('Origin',(110.260001090064,45.5599996354697,380.));
#18101=CARTESIAN_POINT('Origin',(96.5599999999999,35.0599999999999,380.));
#18102=CARTESIAN_POINT('',(98.1601295238092,38.3405617669895,380.));
#18103=CARTESIAN_POINT('',(94.9598704761907,38.3405617669895,380.));
#18104=CARTESIAN_POINT('Origin',(94.9598704761907,38.3405617669895,380.));
#18105=CARTESIAN_POINT('',(93.4240705880017,39.5784009033024,380.));
#18106=CARTESIAN_POINT('Origin',(96.5599999999999,35.0599999999999,380.));
#18107=CARTESIAN_POINT('',(92.0546631075751,38.2146694732975,380.));
#18108=CARTESIAN_POINT('Origin',(92.0546631075751,38.2146694732975,380.));
#18109=CARTESIAN_POINT('Origin',(93.279438268468,33.4598704034959,380.));
#18110=CARTESIAN_POINT('',(92.0546631075751,31.9053305267024,380.));
#18111=CARTESIAN_POINT('Origin',(96.5599999999999,35.0599999999999,380.));
#18112=CARTESIAN_POINT('',(93.4240705880018,30.5415990966974,380.));
#18113=CARTESIAN_POINT('Origin',(93.4240705880018,30.5415990966974,380.));
#18114=CARTESIAN_POINT('',(94.9598704761907,31.7794382330103,380.));
#18115=CARTESIAN_POINT('Origin',(96.5599999999999,35.0599999999999,380.));
#18116=CARTESIAN_POINT('',(98.1601295238092,31.7794382330103,380.));
#18117=CARTESIAN_POINT('Origin',(98.1601295238092,31.7794382330103,380.));
#18118=CARTESIAN_POINT('',(99.6959294119981,30.5415990966974,380.));
#18119=CARTESIAN_POINT('Origin',(96.5599999999999,35.0599999999999,380.));
#18120=CARTESIAN_POINT('',(101.065336892425,31.9053305267024,380.));
#18121=CARTESIAN_POINT('Origin',(101.065336892425,31.9053305267024,380.));
#18122=CARTESIAN_POINT('',(99.8405617315319,33.459870403496,380.));
#18123=CARTESIAN_POINT('Origin',(96.5599999999999,35.0599999999999,380.));
#18124=CARTESIAN_POINT('',(99.8405617315319,36.6601295965039,380.));
#18125=CARTESIAN_POINT('Origin',(99.8405617315319,36.6601295965039,380.));
#18126=CARTESIAN_POINT('',(101.065336892425,38.2146694732975,380.));
#18127=CARTESIAN_POINT('Origin',(96.5599999999999,35.0599999999999,380.));
#18128=CARTESIAN_POINT('',(99.6959294119981,39.5784009033024,380.));
#18129=CARTESIAN_POINT('Origin',(99.6959294119981,39.5784009033024,380.));
#18130=CARTESIAN_POINT('Origin',(83.8599989003778,22.3599995920324,380.));
#18131=CARTESIAN_POINT('',(82.8599989099361,22.3599996015906,380.));
#18132=CARTESIAN_POINT('',(83.859998909936,21.3599996015906,380.));
#18133=CARTESIAN_POINT('Origin',(83.859998909936,21.3599996015906,380.));
#18134=CARTESIAN_POINT('',(86.0599996728755,21.3599996015906,380.));
#18135=CARTESIAN_POINT('Origin',(86.0599996824337,22.3599995920324,380.));
#18136=CARTESIAN_POINT('',(87.0599996728755,22.3599996015906,380.));
#18137=CARTESIAN_POINT('Origin',(87.0599996728755,22.3599996015906,380.));
#18138=CARTESIAN_POINT('',(87.0599996728755,24.5600003645301,380.));
#18139=CARTESIAN_POINT('Origin',(86.0599996824337,24.5600003740883,380.));
#18140=CARTESIAN_POINT('',(86.0599996728755,25.5600003645301,380.));
#18141=CARTESIAN_POINT('Origin',(86.0599996728755,25.5600003645301,380.));
#18142=CARTESIAN_POINT('',(83.859998909936,25.5600003645301,380.));
#18143=CARTESIAN_POINT('Origin',(83.8599989003778,24.5600003740883,380.));
#18144=CARTESIAN_POINT('',(82.8599989099361,24.5600003645301,380.));
#18145=CARTESIAN_POINT('Origin',(82.859998909936,24.5600003645301,380.));
#18146=CARTESIAN_POINT('Origin',(109.260001099622,22.3599995920324,380.));
#18147=CARTESIAN_POINT('',(109.260001090064,21.3599996015906,380.));
#18148=CARTESIAN_POINT('',(110.260001090064,22.3599996015906,380.));
#18149=CARTESIAN_POINT('Origin',(110.260001090064,22.3599996015906,380.));
#18150=CARTESIAN_POINT('',(110.260001090064,24.5600003645301,380.));
#18151=CARTESIAN_POINT('Origin',(109.260001099622,24.5600003740883,380.));
#18152=CARTESIAN_POINT('',(109.260001090064,25.5600003645301,380.));
#18153=CARTESIAN_POINT('Origin',(109.260001090064,25.5600003645301,380.));
#18154=CARTESIAN_POINT('',(107.060000327124,25.5600003645301,380.));
#18155=CARTESIAN_POINT('Origin',(107.060000317566,24.5600003740883,380.));
#18156=CARTESIAN_POINT('',(106.060000327124,24.5600003645301,380.));
#18157=CARTESIAN_POINT('Origin',(106.060000327124,24.5600003645301,380.));
#18158=CARTESIAN_POINT('',(106.060000327124,22.3599996015906,380.));
#18159=CARTESIAN_POINT('Origin',(107.060000317566,22.3599995920324,380.));
#18160=CARTESIAN_POINT('',(107.060000327124,21.3599996015906,380.));
#18161=CARTESIAN_POINT('Origin',(107.060000327124,21.3599996015906,380.));
#18162=CARTESIAN_POINT('Origin',(86.0599996824337,47.7600004079674,380.));
#18163=CARTESIAN_POINT('',(87.0599996728755,47.7600003984092,380.));
#18164=CARTESIAN_POINT('',(86.0599996728755,48.7600003984092,380.));
#18165=CARTESIAN_POINT('Origin',(86.0599996728755,48.7600003984092,380.));
#18166=CARTESIAN_POINT('',(83.859998909936,48.7600003984092,380.));
#18167=CARTESIAN_POINT('Origin',(83.8599989003778,47.7600004079674,380.));
#18168=CARTESIAN_POINT('',(82.8599989099361,47.7600003984092,380.));
#18169=CARTESIAN_POINT('Origin',(82.859998909936,47.7600003984092,380.));
#18170=CARTESIAN_POINT('',(82.8599989099361,45.5599996354697,380.));
#18171=CARTESIAN_POINT('Origin',(83.8599989003778,45.5599996259115,380.));
#18172=CARTESIAN_POINT('',(83.8599989099361,44.5599996354697,380.));
#18173=CARTESIAN_POINT('Origin',(83.8599989099361,44.5599996354697,380.));
#18174=CARTESIAN_POINT('',(86.0599996728755,44.5599996354697,380.));
#18175=CARTESIAN_POINT('Origin',(86.0599996824337,45.5599996259115,380.));
#18176=CARTESIAN_POINT('',(87.0599996728755,45.5599996354697,380.));
#18177=CARTESIAN_POINT('Origin',(87.0599996728755,45.5599996354697,380.));
#18843=UNCERTAINTY_MEASURE_WITH_UNIT(LENGTH_MEASURE(0.01),#18868,
'DISTANCE_ACCURACY_VALUE',
'Maximum model space distance between geometric entities at asserted c
onnectivities');
#18849=UNCERTAINTY_MEASURE_WITH_UNIT(LENGTH_MEASURE(0.01),#18868,
'DISTANCE_ACCURACY_VALUE',
'Maximum model space distance between geometric entities at asserted c
onnectivities');
#18861=(
GEOMETRIC_REPRESENTATION_CONTEXT(3)
GLOBAL_UNCERTAINTY_ASSIGNED_CONTEXT((#18843))
GLOBAL_UNIT_ASSIGNED_CONTEXT((#18868,#18870,#18871))
REPRESENTATION_CONTEXT('','3D')
);
#18867=(
GEOMETRIC_REPRESENTATION_CONTEXT(3)
GLOBAL_UNCERTAINTY_ASSIGNED_CONTEXT((#18849))
GLOBAL_UNIT_ASSIGNED_CONTEXT((#18868,#18870,#18871))
REPRESENTATION_CONTEXT('','3D')
);
#18868=(
LENGTH_UNIT()
NAMED_UNIT(*)
SI_UNIT(.MILLI.,.METRE.)
);
#18870=(
NAMED_UNIT(*)
PLANE_ANGLE_UNIT()
SI_UNIT($,.RADIAN.)
);
#18871=(
NAMED_UNIT(*)
SI_UNIT($,.STERADIAN.)
SOLID_ANGLE_UNIT()
);
#18883=SHAPE_DEFINITION_REPRESENTATION(#18900,#18945);
#18900=PRODUCT_DEFINITION_SHAPE('',$,#18963);
#18945=SHAPE_REPRESENTATION('',(#11712),#18861);
#18951=PRODUCT_DEFINITION_CONTEXT('part definition',#19004,'design');
#18963=PRODUCT_DEFINITION('Frame Side Rail','Frame Side Rail',#18980,#18951);
#18980=PRODUCT_DEFINITION_FORMATION('',$,#19017);
#19004=APPLICATION_CONTEXT(
'Core Data for Automotive Mechanical Design Process');
#19005=PRODUCT_CONTEXT('part definition',#19004,'mechanical');
#19017=PRODUCT('Frame Side Rail','Frame Side Rail',$,(#19005));
#19024=PRESENTATION_STYLE_ASSIGNMENT((#19030));
#19030=SURFACE_STYLE_USAGE(.BOTH.,#19036);
#19036=SURFACE_SIDE_STYLE('',(#19042));
#19042=SURFACE_STYLE_FILL_AREA(#19048);
#19048=FILL_AREA_STYLE('Opaque(20,51,87)',(#19054));
#19054=FILL_AREA_STYLE_COLOUR('Opaque(20,51,87)',#19060);
#19060=COLOUR_RGB('Opaque(20,51,87)',0.0784313725490196,0.2,0.341176470588235);
ENDSEC;
END-ISO-10303-21;
